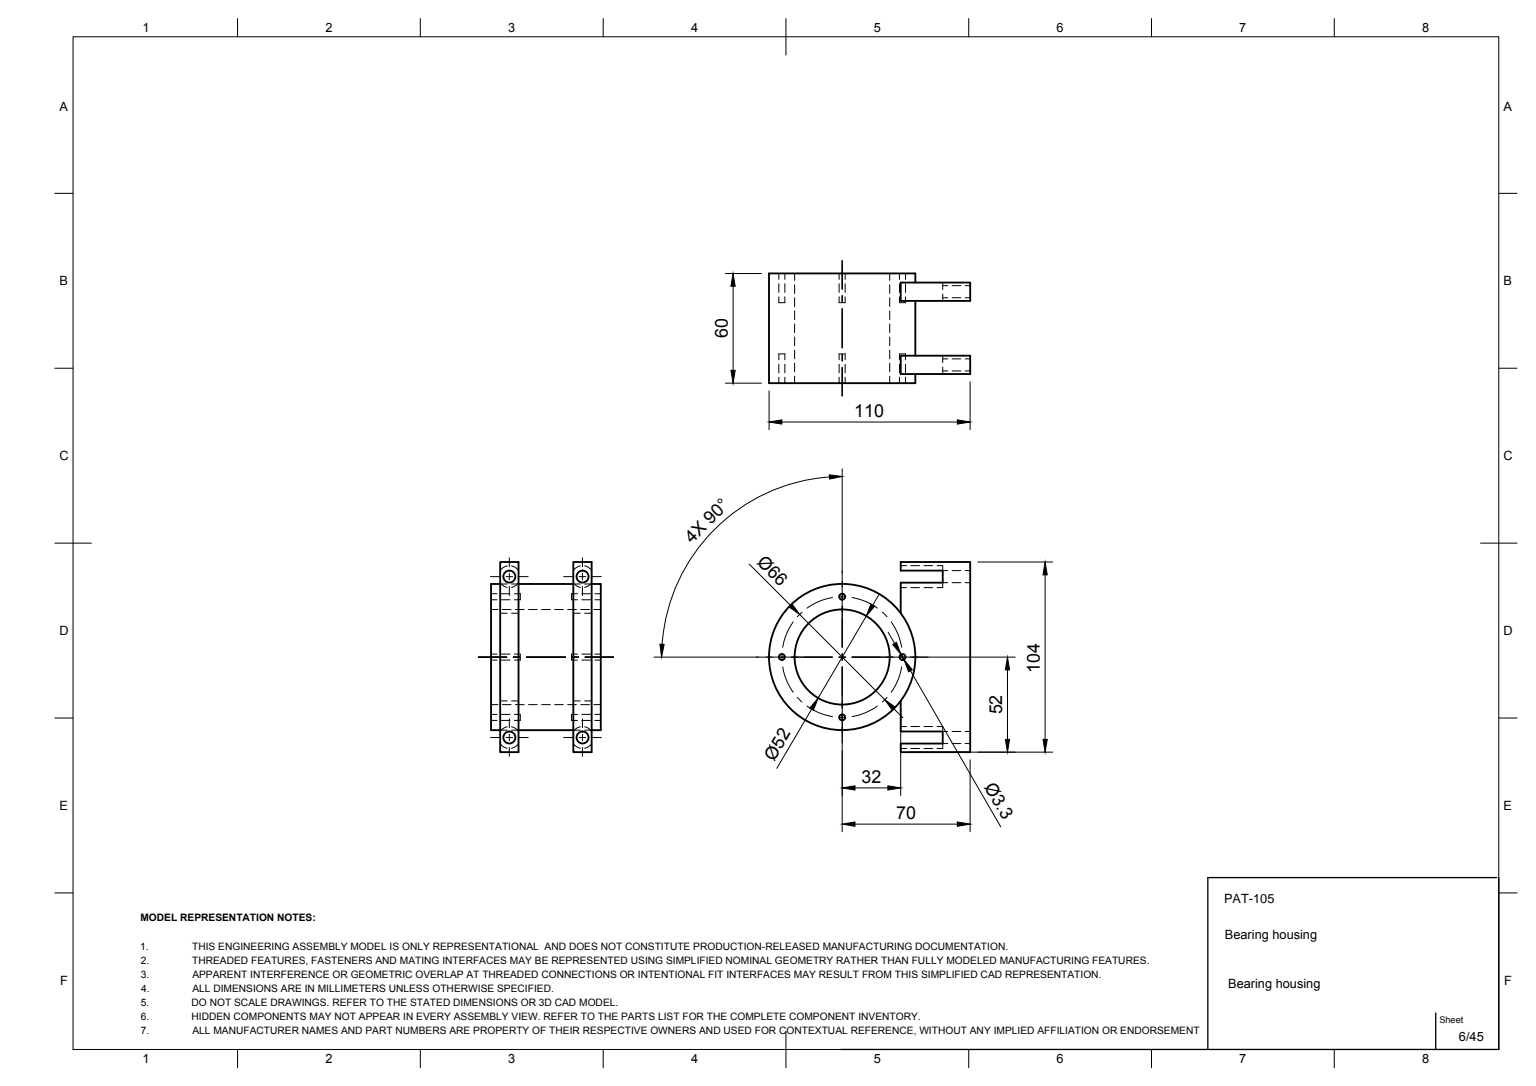
ISO-10303-21;
HEADER;
/* Generated by software containing ST-Developer
 * from STEP Tools, Inc. (www.steptools.com) 
 */

FILE_DESCRIPTION(
/* description */ ('Torque wrench calibration arm'),
/* implementation_level */ '2;1');

FILE_NAME(
/* name */ 'Bearing housing.step',
/* time_stamp */ '2026-10-28T03:24:52-07:00',
/* author */ (''),
/* organization */ (''),
/* preprocessor_version */ 'ST-DEVELOPER v20.2',
/* originating_system */ 'Autodesk Translation Framework v15.17.0.0',
/* authorisation */ '');

FILE_SCHEMA (('AUTOMOTIVE_DESIGN { 1 0 10303 214 3 1 1 }'));
ENDSEC;

DATA;
#10=MECHANICAL_DESIGN_GEOMETRIC_PRESENTATION_REPRESENTATION('',(#427),#12783);
#353=SHAPE_REPRESENTATION_RELATIONSHIP('SRR','None',#12934,#390);
#390=ADVANCED_BREP_SHAPE_REPRESENTATION('',(#481),#12743);
#427=STYLED_ITEM('',(#13212),#481);
#481=MANIFOLD_SOLID_BREP('Body1',#6496);
#539=FACE_BOUND('',#1307,.T.);
#540=FACE_BOUND('',#1311,.T.);
#541=FACE_BOUND('',#1315,.T.);
#542=FACE_BOUND('',#1319,.T.);
#543=FACE_BOUND('',#1336,.T.);
#544=FACE_BOUND('',#1337,.T.);
#545=FACE_BOUND('',#1342,.T.);
#546=FACE_BOUND('',#1343,.T.);
#547=FACE_BOUND('',#1348,.T.);
#548=FACE_BOUND('',#1349,.T.);
#549=FACE_BOUND('',#1351,.T.);
#550=FACE_BOUND('',#1352,.T.);
#551=FACE_BOUND('',#1353,.T.);
#552=FACE_BOUND('',#1354,.T.);
#553=FACE_BOUND('',#1355,.T.);
#554=FACE_BOUND('',#1357,.T.);
#555=FACE_BOUND('',#1358,.T.);
#556=FACE_BOUND('',#1359,.T.);
#557=FACE_BOUND('',#1360,.T.);
#558=FACE_BOUND('',#1361,.T.);
#658=PLANE('',#6985);
#659=PLANE('',#6989);
#660=PLANE('',#6993);
#661=PLANE('',#6997);
#662=PLANE('',#7001);
#663=PLANE('',#7005);
#664=PLANE('',#7009);
#665=PLANE('',#7013);
#666=PLANE('',#7020);
#667=PLANE('',#7028);
#668=PLANE('',#7036);
#669=PLANE('',#7044);
#670=PLANE('',#7046);
#671=PLANE('',#7047);
#672=PLANE('',#7048);
#673=PLANE('',#7049);
#674=PLANE('',#7050);
#675=PLANE('',#7052);
#676=PLANE('',#7053);
#677=PLANE('',#7054);
#678=PLANE('',#7056);
#679=PLANE('',#7057);
#680=PLANE('',#7066);
#681=PLANE('',#7067);
#682=PLANE('',#7068);
#683=PLANE('',#7069);
#684=PLANE('',#7071);
#685=PLANE('',#7072);
#686=PLANE('',#7073);
#687=PLANE('',#7074);
#688=PLANE('',#7082);
#689=PLANE('',#7083);
#885=FACE_OUTER_BOUND('',#1288,.T.);
#886=FACE_OUTER_BOUND('',#1289,.T.);
#887=FACE_OUTER_BOUND('',#1290,.T.);
#888=FACE_OUTER_BOUND('',#1291,.T.);
#889=FACE_OUTER_BOUND('',#1292,.T.);
#890=FACE_OUTER_BOUND('',#1293,.T.);
#891=FACE_OUTER_BOUND('',#1294,.T.);
#892=FACE_OUTER_BOUND('',#1295,.T.);
#893=FACE_OUTER_BOUND('',#1296,.T.);
#894=FACE_OUTER_BOUND('',#1297,.T.);
#895=FACE_OUTER_BOUND('',#1298,.T.);
#896=FACE_OUTER_BOUND('',#1299,.T.);
#897=FACE_OUTER_BOUND('',#1300,.T.);
#898=FACE_OUTER_BOUND('',#1301,.T.);
#899=FACE_OUTER_BOUND('',#1302,.T.);
#900=FACE_OUTER_BOUND('',#1303,.T.);
#901=FACE_OUTER_BOUND('',#1304,.T.);
#902=FACE_OUTER_BOUND('',#1305,.T.);
#903=FACE_OUTER_BOUND('',#1306,.T.);
#904=FACE_OUTER_BOUND('',#1308,.T.);
#905=FACE_OUTER_BOUND('',#1309,.T.);
#906=FACE_OUTER_BOUND('',#1310,.T.);
#907=FACE_OUTER_BOUND('',#1312,.T.);
#908=FACE_OUTER_BOUND('',#1313,.T.);
#909=FACE_OUTER_BOUND('',#1314,.T.);
#910=FACE_OUTER_BOUND('',#1316,.T.);
#911=FACE_OUTER_BOUND('',#1317,.T.);
#912=FACE_OUTER_BOUND('',#1318,.T.);
#913=FACE_OUTER_BOUND('',#1320,.T.);
#914=FACE_OUTER_BOUND('',#1321,.T.);
#915=FACE_OUTER_BOUND('',#1322,.T.);
#916=FACE_OUTER_BOUND('',#1323,.T.);
#917=FACE_OUTER_BOUND('',#1324,.T.);
#918=FACE_OUTER_BOUND('',#1325,.T.);
#919=FACE_OUTER_BOUND('',#1326,.T.);
#920=FACE_OUTER_BOUND('',#1327,.T.);
#921=FACE_OUTER_BOUND('',#1328,.T.);
#922=FACE_OUTER_BOUND('',#1329,.T.);
#923=FACE_OUTER_BOUND('',#1330,.T.);
#924=FACE_OUTER_BOUND('',#1331,.T.);
#925=FACE_OUTER_BOUND('',#1332,.T.);
#926=FACE_OUTER_BOUND('',#1333,.T.);
#927=FACE_OUTER_BOUND('',#1334,.T.);
#928=FACE_OUTER_BOUND('',#1335,.T.);
#929=FACE_OUTER_BOUND('',#1338,.T.);
#930=FACE_OUTER_BOUND('',#1339,.T.);
#931=FACE_OUTER_BOUND('',#1340,.T.);
#932=FACE_OUTER_BOUND('',#1341,.T.);
#933=FACE_OUTER_BOUND('',#1344,.T.);
#934=FACE_OUTER_BOUND('',#1345,.T.);
#935=FACE_OUTER_BOUND('',#1346,.T.);
#936=FACE_OUTER_BOUND('',#1347,.T.);
#937=FACE_OUTER_BOUND('',#1350,.T.);
#938=FACE_OUTER_BOUND('',#1356,.T.);
#1288=EDGE_LOOP('',(#4399,#4400,#4401,#4402));
#1289=EDGE_LOOP('',(#4403));
#1290=EDGE_LOOP('',(#4404,#4405,#4406,#4407));
#1291=EDGE_LOOP('',(#4408));
#1292=EDGE_LOOP('',(#4409,#4410,#4411,#4412));
#1293=EDGE_LOOP('',(#4413));
#1294=EDGE_LOOP('',(#4414,#4415,#4416,#4417));
#1295=EDGE_LOOP('',(#4418));
#1296=EDGE_LOOP('',(#4419,#4420,#4421,#4422));
#1297=EDGE_LOOP('',(#4423));
#1298=EDGE_LOOP('',(#4424,#4425,#4426,#4427));
#1299=EDGE_LOOP('',(#4428));
#1300=EDGE_LOOP('',(#4429,#4430,#4431,#4432));
#1301=EDGE_LOOP('',(#4433));
#1302=EDGE_LOOP('',(#4434,#4435,#4436,#4437));
#1303=EDGE_LOOP('',(#4438));
#1304=EDGE_LOOP('',(#4439,#4440,#4441,#4442));
#1305=EDGE_LOOP('',(#4443,#4444,#4445,#4446));
#1306=EDGE_LOOP('',(#4447,#4448,#4449,#4450));
#1307=EDGE_LOOP('',(#4451));
#1308=EDGE_LOOP('',(#4452,#4453,#4454,#4455));
#1309=EDGE_LOOP('',(#4456,#4457,#4458,#4459));
#1310=EDGE_LOOP('',(#4460,#4461,#4462,#4463));
#1311=EDGE_LOOP('',(#4464));
#1312=EDGE_LOOP('',(#4465,#4466,#4467,#4468));
#1313=EDGE_LOOP('',(#4469,#4470,#4471,#4472));
#1314=EDGE_LOOP('',(#4473,#4474,#4475,#4476));
#1315=EDGE_LOOP('',(#4477));
#1316=EDGE_LOOP('',(#4478,#4479,#4480,#4481));
#1317=EDGE_LOOP('',(#4482,#4483,#4484,#4485));
#1318=EDGE_LOOP('',(#4486,#4487,#4488,#4489));
#1319=EDGE_LOOP('',(#4490));
#1320=EDGE_LOOP('',(#4491,#4492,#4493,#4494));
#1321=EDGE_LOOP('',(#4495,#4496,#4497,#4498));
#1322=EDGE_LOOP('',(#4499,#4500,#4501,#4502));
#1323=EDGE_LOOP('',(#4503,#4504,#4505,#4506));
#1324=EDGE_LOOP('',(#4507,#4508,#4509,#4510,#4511,#4512,#4513,#4514,#4515,
#4516,#4517,#4518,#4519,#4520));
#1325=EDGE_LOOP('',(#4521,#4522,#4523,#4524));
#1326=EDGE_LOOP('',(#4525,#4526,#4527,#4528));
#1327=EDGE_LOOP('',(#4529,#4530,#4531,#4532,#4533,#4534,#4535,#4536,#4537,
#4538,#4539,#4540,#4541,#4542));
#1328=EDGE_LOOP('',(#4543,#4544,#4545,#4546));
#1329=EDGE_LOOP('',(#4547,#4548,#4549,#4550));
#1330=EDGE_LOOP('',(#4551,#4552,#4553,#4554));
#1331=EDGE_LOOP('',(#4555,#4556,#4557,#4558));
#1332=EDGE_LOOP('',(#4559,#4560,#4561,#4562));
#1333=EDGE_LOOP('',(#4563,#4564,#4565,#4566));
#1334=EDGE_LOOP('',(#4567,#4568,#4569,#4570));
#1335=EDGE_LOOP('',(#4571,#4572,#4573,#4574));
#1336=EDGE_LOOP('',(#4575));
#1337=EDGE_LOOP('',(#4576));
#1338=EDGE_LOOP('',(#4577,#4578,#4579,#4580));
#1339=EDGE_LOOP('',(#4581,#4582,#4583,#4584,#4585,#4586,#4587,#4588,#4589,
#4590,#4591,#4592,#4593,#4594));
#1340=EDGE_LOOP('',(#4595,#4596,#4597,#4598));
#1341=EDGE_LOOP('',(#4599,#4600,#4601,#4602));
#1342=EDGE_LOOP('',(#4603));
#1343=EDGE_LOOP('',(#4604));
#1344=EDGE_LOOP('',(#4605,#4606,#4607,#4608));
#1345=EDGE_LOOP('',(#4609,#4610,#4611,#4612,#4613,#4614,#4615,#4616,#4617,
#4618,#4619,#4620,#4621,#4622));
#1346=EDGE_LOOP('',(#4623,#4624,#4625,#4626));
#1347=EDGE_LOOP('',(#4627,#4628,#4629,#4630));
#1348=EDGE_LOOP('',(#4631,#4632,#4633,#4634));
#1349=EDGE_LOOP('',(#4635,#4636,#4637,#4638));
#1350=EDGE_LOOP('',(#4639));
#1351=EDGE_LOOP('',(#4640));
#1352=EDGE_LOOP('',(#4641));
#1353=EDGE_LOOP('',(#4642));
#1354=EDGE_LOOP('',(#4643));
#1355=EDGE_LOOP('',(#4644));
#1356=EDGE_LOOP('',(#4645));
#1357=EDGE_LOOP('',(#4646));
#1358=EDGE_LOOP('',(#4647));
#1359=EDGE_LOOP('',(#4648));
#1360=EDGE_LOOP('',(#4649));
#1361=EDGE_LOOP('',(#4650));
#1802=LINE('',#9983,#2217);
#1803=LINE('',#9990,#2218);
#1804=LINE('',#9997,#2219);
#1805=LINE('',#10004,#2220);
#1806=LINE('',#10011,#2221);
#1807=LINE('',#10018,#2222);
#1808=LINE('',#10025,#2223);
#1809=LINE('',#10032,#2224);
#1810=LINE('',#10038,#2225);
#1811=LINE('',#10042,#2226);
#1812=LINE('',#10047,#2227);
#1813=LINE('',#10051,#2228);
#1814=LINE('',#10054,#2229);
#1815=LINE('',#10055,#2230);
#1816=LINE('',#10061,#2231);
#1817=LINE('',#10065,#2232);
#1818=LINE('',#10070,#2233);
#1819=LINE('',#10074,#2234);
#1820=LINE('',#10077,#2235);
#1821=LINE('',#10078,#2236);
#1822=LINE('',#10084,#2237);
#1823=LINE('',#10088,#2238);
#1824=LINE('',#10093,#2239);
#1825=LINE('',#10097,#2240);
#1826=LINE('',#10100,#2241);
#1827=LINE('',#10101,#2242);
#1828=LINE('',#10107,#2243);
#1829=LINE('',#10111,#2244);
#1830=LINE('',#10116,#2245);
#1831=LINE('',#10120,#2246);
#1832=LINE('',#10123,#2247);
#1833=LINE('',#10124,#2248);
#1834=LINE('',#10129,#2249);
#1835=LINE('',#10131,#2250);
#1836=LINE('',#10132,#2251);
#1837=LINE('',#10135,#2252);
#1838=LINE('',#10137,#2253);
#1839=LINE('',#10138,#2254);
#1840=LINE('',#10141,#2255);
#1841=LINE('',#10143,#2256);
#1842=LINE('',#10144,#2257);
#1843=LINE('',#10147,#2258);
#1844=LINE('',#10149,#2259);
#1845=LINE('',#10150,#2260);
#1846=LINE('',#10153,#2261);
#1847=LINE('',#10155,#2262);
#1848=LINE('',#10157,#2263);
#1849=LINE('',#10158,#2264);
#1850=LINE('',#10160,#2265);
#1851=LINE('',#10164,#2266);
#1852=LINE('',#10165,#2267);
#1853=LINE('',#10168,#2268);
#1854=LINE('',#10169,#2269);
#1855=LINE('',#10173,#2270);
#1856=LINE('',#10175,#2271);
#1857=LINE('',#10177,#2272);
#1858=LINE('',#10179,#2273);
#1859=LINE('',#10180,#2274);
#1860=LINE('',#10183,#2275);
#1861=LINE('',#10184,#2276);
#1862=LINE('',#10187,#2277);
#1863=LINE('',#10188,#2278);
#1864=LINE('',#10192,#2279);
#1865=LINE('',#10196,#2280);
#1866=LINE('',#10200,#2281);
#1867=LINE('',#10204,#2282);
#1868=LINE('',#10207,#2283);
#1869=LINE('',#10208,#2284);
#1870=LINE('',#10211,#2285);
#1871=LINE('',#10212,#2286);
#1872=LINE('',#10214,#2287);
#1873=LINE('',#10219,#2288);
#1874=LINE('',#10220,#2289);
#1875=LINE('',#10223,#2290);
#1876=LINE('',#10224,#2291);
#1877=LINE('',#10226,#2292);
#1878=LINE('',#10233,#2293);
#1879=LINE('',#10239,#2294);
#2217=VECTOR('',#7874,0.165);
#2218=VECTOR('',#7883,0.165);
#2219=VECTOR('',#7892,0.165);
#2220=VECTOR('',#7901,0.165);
#2221=VECTOR('',#7910,0.165);
#2222=VECTOR('',#7919,0.165);
#2223=VECTOR('',#7928,0.165);
#2224=VECTOR('',#7937,0.165);
#2225=VECTOR('',#7944,1.);
#2226=VECTOR('',#7947,1.);
#2227=VECTOR('',#7952,1.);
#2228=VECTOR('',#7955,1.);
#2229=VECTOR('',#7960,1.);
#2230=VECTOR('',#7961,1.);
#2231=VECTOR('',#7966,1.);
#2232=VECTOR('',#7969,1.);
#2233=VECTOR('',#7974,1.);
#2234=VECTOR('',#7977,1.);
#2235=VECTOR('',#7982,1.);
#2236=VECTOR('',#7983,1.);
#2237=VECTOR('',#7988,1.);
#2238=VECTOR('',#7991,1.);
#2239=VECTOR('',#7996,1.);
#2240=VECTOR('',#7999,1.);
#2241=VECTOR('',#8004,1.);
#2242=VECTOR('',#8005,1.);
#2243=VECTOR('',#8010,1.);
#2244=VECTOR('',#8013,1.);
#2245=VECTOR('',#8018,1.);
#2246=VECTOR('',#8021,1.);
#2247=VECTOR('',#8026,1.);
#2248=VECTOR('',#8027,1.);
#2249=VECTOR('',#8032,1.);
#2250=VECTOR('',#8033,1.);
#2251=VECTOR('',#8034,1.);
#2252=VECTOR('',#8037,1.);
#2253=VECTOR('',#8038,1.);
#2254=VECTOR('',#8039,1.);
#2255=VECTOR('',#8042,1.);
#2256=VECTOR('',#8043,1.);
#2257=VECTOR('',#8044,1.);
#2258=VECTOR('',#8047,1.);
#2259=VECTOR('',#8048,1.);
#2260=VECTOR('',#8049,1.);
#2261=VECTOR('',#8052,1.);
#2262=VECTOR('',#8053,1.);
#2263=VECTOR('',#8054,1.);
#2264=VECTOR('',#8055,1.);
#2265=VECTOR('',#8056,1.);
#2266=VECTOR('',#8061,1.);
#2267=VECTOR('',#8062,1.);
#2268=VECTOR('',#8065,1.);
#2269=VECTOR('',#8066,1.);
#2270=VECTOR('',#8071,1.);
#2271=VECTOR('',#8072,1.);
#2272=VECTOR('',#8073,1.);
#2273=VECTOR('',#8074,1.);
#2274=VECTOR('',#8075,1.);
#2275=VECTOR('',#8078,1.);
#2276=VECTOR('',#8079,1.);
#2277=VECTOR('',#8082,1.);
#2278=VECTOR('',#8083,1.);
#2279=VECTOR('',#8088,0.33);
#2280=VECTOR('',#8093,0.33);
#2281=VECTOR('',#8098,0.33);
#2282=VECTOR('',#8103,0.33);
#2283=VECTOR('',#8106,1.);
#2284=VECTOR('',#8107,1.);
#2285=VECTOR('',#8110,1.);
#2286=VECTOR('',#8111,1.);
#2287=VECTOR('',#8114,1.);
#2288=VECTOR('',#8121,1.);
#2289=VECTOR('',#8122,1.);
#2290=VECTOR('',#8125,1.);
#2291=VECTOR('',#8126,1.);
#2292=VECTOR('',#8129,1.);
#2293=VECTOR('',#8138,2.6);
#2294=VECTOR('',#8145,4.);
#2624=CIRCLE('',#6983,0.165);
#2625=CIRCLE('',#6984,0.165);
#2626=CIRCLE('',#6987,0.165);
#2627=CIRCLE('',#6988,0.165);
#2628=CIRCLE('',#6991,0.165);
#2629=CIRCLE('',#6992,0.165);
#2630=CIRCLE('',#6995,0.165);
#2631=CIRCLE('',#6996,0.165);
#2632=CIRCLE('',#6999,0.165);
#2633=CIRCLE('',#7000,0.165);
#2634=CIRCLE('',#7003,0.165);
#2635=CIRCLE('',#7004,0.165);
#2636=CIRCLE('',#7007,0.165);
#2637=CIRCLE('',#7008,0.165);
#2638=CIRCLE('',#7011,0.165);
#2639=CIRCLE('',#7012,0.165);
#2640=CIRCLE('',#7015,0.6);
#2641=CIRCLE('',#7016,0.6);
#2642=CIRCLE('',#7018,0.6);
#2643=CIRCLE('',#7019,0.6);
#2644=CIRCLE('',#7021,0.33);
#2645=CIRCLE('',#7023,0.6);
#2646=CIRCLE('',#7024,0.6);
#2647=CIRCLE('',#7026,0.6);
#2648=CIRCLE('',#7027,0.6);
#2649=CIRCLE('',#7029,0.33);
#2650=CIRCLE('',#7031,0.6);
#2651=CIRCLE('',#7032,0.6);
#2652=CIRCLE('',#7034,0.6);
#2653=CIRCLE('',#7035,0.6);
#2654=CIRCLE('',#7037,0.33);
#2655=CIRCLE('',#7039,0.6);
#2656=CIRCLE('',#7040,0.6);
#2657=CIRCLE('',#7042,0.6);
#2658=CIRCLE('',#7043,0.6);
#2659=CIRCLE('',#7045,0.33);
#2660=CIRCLE('',#7051,4.);
#2661=CIRCLE('',#7055,4.);
#2662=CIRCLE('',#7059,0.33);
#2663=CIRCLE('',#7061,0.33);
#2664=CIRCLE('',#7063,0.33);
#2665=CIRCLE('',#7065,0.33);
#2666=CIRCLE('',#7070,4.);
#2667=CIRCLE('',#7075,4.);
#2668=CIRCLE('',#7077,2.6);
#2669=CIRCLE('',#7078,2.6);
#2670=CIRCLE('',#7080,4.);
#2671=CIRCLE('',#7081,4.);
#2987=VERTEX_POINT('',#9980);
#2988=VERTEX_POINT('',#9982);
#2989=VERTEX_POINT('',#9987);
#2990=VERTEX_POINT('',#9989);
#2991=VERTEX_POINT('',#9994);
#2992=VERTEX_POINT('',#9996);
#2993=VERTEX_POINT('',#10001);
#2994=VERTEX_POINT('',#10003);
#2995=VERTEX_POINT('',#10008);
#2996=VERTEX_POINT('',#10010);
#2997=VERTEX_POINT('',#10015);
#2998=VERTEX_POINT('',#10017);
#2999=VERTEX_POINT('',#10022);
#3000=VERTEX_POINT('',#10024);
#3001=VERTEX_POINT('',#10029);
#3002=VERTEX_POINT('',#10031);
#3003=VERTEX_POINT('',#10036);
#3004=VERTEX_POINT('',#10037);
#3005=VERTEX_POINT('',#10039);
#3006=VERTEX_POINT('',#10041);
#3007=VERTEX_POINT('',#10045);
#3008=VERTEX_POINT('',#10046);
#3009=VERTEX_POINT('',#10048);
#3010=VERTEX_POINT('',#10050);
#3011=VERTEX_POINT('',#10056);
#3012=VERTEX_POINT('',#10059);
#3013=VERTEX_POINT('',#10060);
#3014=VERTEX_POINT('',#10062);
#3015=VERTEX_POINT('',#10064);
#3016=VERTEX_POINT('',#10068);
#3017=VERTEX_POINT('',#10069);
#3018=VERTEX_POINT('',#10071);
#3019=VERTEX_POINT('',#10073);
#3020=VERTEX_POINT('',#10079);
#3021=VERTEX_POINT('',#10082);
#3022=VERTEX_POINT('',#10083);
#3023=VERTEX_POINT('',#10085);
#3024=VERTEX_POINT('',#10087);
#3025=VERTEX_POINT('',#10091);
#3026=VERTEX_POINT('',#10092);
#3027=VERTEX_POINT('',#10094);
#3028=VERTEX_POINT('',#10096);
#3029=VERTEX_POINT('',#10102);
#3030=VERTEX_POINT('',#10105);
#3031=VERTEX_POINT('',#10106);
#3032=VERTEX_POINT('',#10108);
#3033=VERTEX_POINT('',#10110);
#3034=VERTEX_POINT('',#10114);
#3035=VERTEX_POINT('',#10115);
#3036=VERTEX_POINT('',#10117);
#3037=VERTEX_POINT('',#10119);
#3038=VERTEX_POINT('',#10125);
#3039=VERTEX_POINT('',#10128);
#3040=VERTEX_POINT('',#10130);
#3041=VERTEX_POINT('',#10134);
#3042=VERTEX_POINT('',#10136);
#3043=VERTEX_POINT('',#10140);
#3044=VERTEX_POINT('',#10142);
#3045=VERTEX_POINT('',#10146);
#3046=VERTEX_POINT('',#10148);
#3047=VERTEX_POINT('',#10152);
#3048=VERTEX_POINT('',#10154);
#3049=VERTEX_POINT('',#10156);
#3050=VERTEX_POINT('',#10159);
#3051=VERTEX_POINT('',#10163);
#3052=VERTEX_POINT('',#10167);
#3053=VERTEX_POINT('',#10171);
#3054=VERTEX_POINT('',#10174);
#3055=VERTEX_POINT('',#10176);
#3056=VERTEX_POINT('',#10178);
#3057=VERTEX_POINT('',#10182);
#3058=VERTEX_POINT('',#10186);
#3059=VERTEX_POINT('',#10190);
#3060=VERTEX_POINT('',#10194);
#3061=VERTEX_POINT('',#10198);
#3062=VERTEX_POINT('',#10202);
#3063=VERTEX_POINT('',#10206);
#3064=VERTEX_POINT('',#10210);
#3065=VERTEX_POINT('',#10218);
#3066=VERTEX_POINT('',#10222);
#3067=VERTEX_POINT('',#10230);
#3068=VERTEX_POINT('',#10232);
#3069=VERTEX_POINT('',#10236);
#3070=VERTEX_POINT('',#10238);
#3557=EDGE_CURVE('',#2987,#2987,#2624,.T.);
#3558=EDGE_CURVE('',#2987,#2988,#1802,.T.);
#3559=EDGE_CURVE('',#2988,#2988,#2625,.T.);
#3560=EDGE_CURVE('',#2989,#2989,#2626,.T.);
#3561=EDGE_CURVE('',#2989,#2990,#1803,.T.);
#3562=EDGE_CURVE('',#2990,#2990,#2627,.T.);
#3563=EDGE_CURVE('',#2991,#2991,#2628,.T.);
#3564=EDGE_CURVE('',#2991,#2992,#1804,.T.);
#3565=EDGE_CURVE('',#2992,#2992,#2629,.T.);
#3566=EDGE_CURVE('',#2993,#2993,#2630,.T.);
#3567=EDGE_CURVE('',#2993,#2994,#1805,.T.);
#3568=EDGE_CURVE('',#2994,#2994,#2631,.T.);
#3569=EDGE_CURVE('',#2995,#2995,#2632,.T.);
#3570=EDGE_CURVE('',#2995,#2996,#1806,.T.);
#3571=EDGE_CURVE('',#2996,#2996,#2633,.T.);
#3572=EDGE_CURVE('',#2997,#2997,#2634,.T.);
#3573=EDGE_CURVE('',#2997,#2998,#1807,.T.);
#3574=EDGE_CURVE('',#2998,#2998,#2635,.T.);
#3575=EDGE_CURVE('',#2999,#2999,#2636,.T.);
#3576=EDGE_CURVE('',#2999,#3000,#1808,.T.);
#3577=EDGE_CURVE('',#3000,#3000,#2637,.T.);
#3578=EDGE_CURVE('',#3001,#3001,#2638,.T.);
#3579=EDGE_CURVE('',#3001,#3002,#1809,.T.);
#3580=EDGE_CURVE('',#3002,#3002,#2639,.T.);
#3581=EDGE_CURVE('',#3003,#3004,#1810,.T.);
#3582=EDGE_CURVE('',#3005,#3003,#2640,.T.);
#3583=EDGE_CURVE('',#3006,#3005,#1811,.T.);
#3584=EDGE_CURVE('',#3004,#3006,#2641,.T.);
#3585=EDGE_CURVE('',#3007,#3008,#1812,.T.);
#3586=EDGE_CURVE('',#3009,#3007,#2642,.T.);
#3587=EDGE_CURVE('',#3010,#3009,#1813,.T.);
#3588=EDGE_CURVE('',#3008,#3010,#2643,.T.);
#3589=EDGE_CURVE('',#3004,#3007,#1814,.T.);
#3590=EDGE_CURVE('',#3009,#3006,#1815,.T.);
#3591=EDGE_CURVE('',#3011,#3011,#2644,.T.);
#3592=EDGE_CURVE('',#3012,#3013,#1816,.T.);
#3593=EDGE_CURVE('',#3014,#3012,#2645,.T.);
#3594=EDGE_CURVE('',#3015,#3014,#1817,.T.);
#3595=EDGE_CURVE('',#3013,#3015,#2646,.T.);
#3596=EDGE_CURVE('',#3016,#3017,#1818,.T.);
#3597=EDGE_CURVE('',#3018,#3016,#2647,.T.);
#3598=EDGE_CURVE('',#3019,#3018,#1819,.T.);
#3599=EDGE_CURVE('',#3017,#3019,#2648,.T.);
#3600=EDGE_CURVE('',#3013,#3016,#1820,.T.);
#3601=EDGE_CURVE('',#3018,#3015,#1821,.T.);
#3602=EDGE_CURVE('',#3020,#3020,#2649,.T.);
#3603=EDGE_CURVE('',#3021,#3022,#1822,.T.);
#3604=EDGE_CURVE('',#3023,#3021,#2650,.T.);
#3605=EDGE_CURVE('',#3024,#3023,#1823,.T.);
#3606=EDGE_CURVE('',#3022,#3024,#2651,.T.);
#3607=EDGE_CURVE('',#3025,#3026,#1824,.T.);
#3608=EDGE_CURVE('',#3027,#3025,#2652,.T.);
#3609=EDGE_CURVE('',#3028,#3027,#1825,.T.);
#3610=EDGE_CURVE('',#3026,#3028,#2653,.T.);
#3611=EDGE_CURVE('',#3022,#3025,#1826,.T.);
#3612=EDGE_CURVE('',#3027,#3024,#1827,.T.);
#3613=EDGE_CURVE('',#3029,#3029,#2654,.T.);
#3614=EDGE_CURVE('',#3030,#3031,#1828,.T.);
#3615=EDGE_CURVE('',#3032,#3030,#2655,.T.);
#3616=EDGE_CURVE('',#3033,#3032,#1829,.T.);
#3617=EDGE_CURVE('',#3031,#3033,#2656,.T.);
#3618=EDGE_CURVE('',#3034,#3035,#1830,.T.);
#3619=EDGE_CURVE('',#3036,#3034,#2657,.T.);
#3620=EDGE_CURVE('',#3037,#3036,#1831,.T.);
#3621=EDGE_CURVE('',#3035,#3037,#2658,.T.);
#3622=EDGE_CURVE('',#3031,#3034,#1832,.T.);
#3623=EDGE_CURVE('',#3036,#3033,#1833,.T.);
#3624=EDGE_CURVE('',#3038,#3038,#2659,.T.);
#3625=EDGE_CURVE('',#3039,#3003,#1834,.T.);
#3626=EDGE_CURVE('',#3039,#3040,#1835,.T.);
#3627=EDGE_CURVE('',#3005,#3040,#1836,.T.);
#3628=EDGE_CURVE('',#3041,#3010,#1837,.T.);
#3629=EDGE_CURVE('',#3042,#3041,#1838,.T.);
#3630=EDGE_CURVE('',#3008,#3042,#1839,.T.);
#3631=EDGE_CURVE('',#3043,#3012,#1840,.T.);
#3632=EDGE_CURVE('',#3044,#3043,#1841,.T.);
#3633=EDGE_CURVE('',#3014,#3044,#1842,.T.);
#3634=EDGE_CURVE('',#3045,#3019,#1843,.T.);
#3635=EDGE_CURVE('',#3046,#3045,#1844,.T.);
#3636=EDGE_CURVE('',#3017,#3046,#1845,.T.);
#3637=EDGE_CURVE('',#3040,#3047,#1846,.T.);
#3638=EDGE_CURVE('',#3047,#3048,#1847,.T.);
#3639=EDGE_CURVE('',#3048,#3049,#1848,.T.);
#3640=EDGE_CURVE('',#3049,#3028,#1849,.T.);
#3641=EDGE_CURVE('',#3023,#3050,#1850,.T.);
#3642=EDGE_CURVE('',#3041,#3050,#2660,.T.);
#3643=EDGE_CURVE('',#3051,#3021,#1851,.T.);
#3644=EDGE_CURVE('',#3050,#3051,#1852,.T.);
#3645=EDGE_CURVE('',#3052,#3049,#1853,.T.);
#3646=EDGE_CURVE('',#3026,#3052,#1854,.T.);
#3647=EDGE_CURVE('',#3053,#3044,#2661,.T.);
#3648=EDGE_CURVE('',#3053,#3037,#1855,.T.);
#3649=EDGE_CURVE('',#3032,#3054,#1856,.T.);
#3650=EDGE_CURVE('',#3054,#3055,#1857,.T.);
#3651=EDGE_CURVE('',#3055,#3056,#1858,.T.);
#3652=EDGE_CURVE('',#3056,#3045,#1859,.T.);
#3653=EDGE_CURVE('',#3057,#3030,#1860,.T.);
#3654=EDGE_CURVE('',#3057,#3054,#1861,.T.);
#3655=EDGE_CURVE('',#3058,#3053,#1862,.T.);
#3656=EDGE_CURVE('',#3035,#3058,#1863,.T.);
#3657=EDGE_CURVE('',#3059,#3059,#2662,.T.);
#3658=EDGE_CURVE('',#3059,#3011,#1864,.T.);
#3659=EDGE_CURVE('',#3060,#3060,#2663,.T.);
#3660=EDGE_CURVE('',#3060,#3020,#1865,.T.);
#3661=EDGE_CURVE('',#3061,#3061,#2664,.T.);
#3662=EDGE_CURVE('',#3061,#3029,#1866,.T.);
#3663=EDGE_CURVE('',#3062,#3062,#2665,.T.);
#3664=EDGE_CURVE('',#3062,#3038,#1867,.T.);
#3665=EDGE_CURVE('',#3046,#3063,#1868,.T.);
#3666=EDGE_CURVE('',#3063,#3056,#1869,.T.);
#3667=EDGE_CURVE('',#3063,#3064,#1870,.T.);
#3668=EDGE_CURVE('',#3064,#3055,#1871,.T.);
#3669=EDGE_CURVE('',#3064,#3057,#1872,.T.);
#3670=EDGE_CURVE('',#3043,#3058,#2666,.T.);
#3671=EDGE_CURVE('',#3052,#3065,#1873,.T.);
#3672=EDGE_CURVE('',#3065,#3048,#1874,.T.);
#3673=EDGE_CURVE('',#3065,#3066,#1875,.T.);
#3674=EDGE_CURVE('',#3066,#3047,#1876,.T.);
#3675=EDGE_CURVE('',#3066,#3039,#1877,.T.);
#3676=EDGE_CURVE('',#3051,#3042,#2667,.T.);
#3677=EDGE_CURVE('',#3067,#3067,#2668,.T.);
#3678=EDGE_CURVE('',#3067,#3068,#1878,.T.);
#3679=EDGE_CURVE('',#3068,#3068,#2669,.T.);
#3680=EDGE_CURVE('',#3069,#3069,#2670,.T.);
#3681=EDGE_CURVE('',#3069,#3070,#1879,.T.);
#3682=EDGE_CURVE('',#3070,#3070,#2671,.T.);
#4399=ORIENTED_EDGE('',*,*,#3557,.F.);
#4400=ORIENTED_EDGE('',*,*,#3558,.T.);
#4401=ORIENTED_EDGE('',*,*,#3559,.F.);
#4402=ORIENTED_EDGE('',*,*,#3558,.F.);
#4403=ORIENTED_EDGE('',*,*,#3557,.T.);
#4404=ORIENTED_EDGE('',*,*,#3560,.F.);
#4405=ORIENTED_EDGE('',*,*,#3561,.T.);
#4406=ORIENTED_EDGE('',*,*,#3562,.F.);
#4407=ORIENTED_EDGE('',*,*,#3561,.F.);
#4408=ORIENTED_EDGE('',*,*,#3560,.T.);
#4409=ORIENTED_EDGE('',*,*,#3563,.F.);
#4410=ORIENTED_EDGE('',*,*,#3564,.T.);
#4411=ORIENTED_EDGE('',*,*,#3565,.F.);
#4412=ORIENTED_EDGE('',*,*,#3564,.F.);
#4413=ORIENTED_EDGE('',*,*,#3563,.T.);
#4414=ORIENTED_EDGE('',*,*,#3566,.F.);
#4415=ORIENTED_EDGE('',*,*,#3567,.T.);
#4416=ORIENTED_EDGE('',*,*,#3568,.F.);
#4417=ORIENTED_EDGE('',*,*,#3567,.F.);
#4418=ORIENTED_EDGE('',*,*,#3566,.T.);
#4419=ORIENTED_EDGE('',*,*,#3569,.F.);
#4420=ORIENTED_EDGE('',*,*,#3570,.T.);
#4421=ORIENTED_EDGE('',*,*,#3571,.T.);
#4422=ORIENTED_EDGE('',*,*,#3570,.F.);
#4423=ORIENTED_EDGE('',*,*,#3571,.F.);
#4424=ORIENTED_EDGE('',*,*,#3572,.F.);
#4425=ORIENTED_EDGE('',*,*,#3573,.T.);
#4426=ORIENTED_EDGE('',*,*,#3574,.T.);
#4427=ORIENTED_EDGE('',*,*,#3573,.F.);
#4428=ORIENTED_EDGE('',*,*,#3574,.F.);
#4429=ORIENTED_EDGE('',*,*,#3575,.F.);
#4430=ORIENTED_EDGE('',*,*,#3576,.T.);
#4431=ORIENTED_EDGE('',*,*,#3577,.T.);
#4432=ORIENTED_EDGE('',*,*,#3576,.F.);
#4433=ORIENTED_EDGE('',*,*,#3577,.F.);
#4434=ORIENTED_EDGE('',*,*,#3578,.F.);
#4435=ORIENTED_EDGE('',*,*,#3579,.T.);
#4436=ORIENTED_EDGE('',*,*,#3580,.T.);
#4437=ORIENTED_EDGE('',*,*,#3579,.F.);
#4438=ORIENTED_EDGE('',*,*,#3580,.F.);
#4439=ORIENTED_EDGE('',*,*,#3581,.F.);
#4440=ORIENTED_EDGE('',*,*,#3582,.F.);
#4441=ORIENTED_EDGE('',*,*,#3583,.F.);
#4442=ORIENTED_EDGE('',*,*,#3584,.F.);
#4443=ORIENTED_EDGE('',*,*,#3585,.F.);
#4444=ORIENTED_EDGE('',*,*,#3586,.F.);
#4445=ORIENTED_EDGE('',*,*,#3587,.F.);
#4446=ORIENTED_EDGE('',*,*,#3588,.F.);
#4447=ORIENTED_EDGE('',*,*,#3589,.F.);
#4448=ORIENTED_EDGE('',*,*,#3584,.T.);
#4449=ORIENTED_EDGE('',*,*,#3590,.F.);
#4450=ORIENTED_EDGE('',*,*,#3586,.T.);
#4451=ORIENTED_EDGE('',*,*,#3591,.F.);
#4452=ORIENTED_EDGE('',*,*,#3592,.F.);
#4453=ORIENTED_EDGE('',*,*,#3593,.F.);
#4454=ORIENTED_EDGE('',*,*,#3594,.F.);
#4455=ORIENTED_EDGE('',*,*,#3595,.F.);
#4456=ORIENTED_EDGE('',*,*,#3596,.F.);
#4457=ORIENTED_EDGE('',*,*,#3597,.F.);
#4458=ORIENTED_EDGE('',*,*,#3598,.F.);
#4459=ORIENTED_EDGE('',*,*,#3599,.F.);
#4460=ORIENTED_EDGE('',*,*,#3600,.F.);
#4461=ORIENTED_EDGE('',*,*,#3595,.T.);
#4462=ORIENTED_EDGE('',*,*,#3601,.F.);
#4463=ORIENTED_EDGE('',*,*,#3597,.T.);
#4464=ORIENTED_EDGE('',*,*,#3602,.F.);
#4465=ORIENTED_EDGE('',*,*,#3603,.F.);
#4466=ORIENTED_EDGE('',*,*,#3604,.F.);
#4467=ORIENTED_EDGE('',*,*,#3605,.F.);
#4468=ORIENTED_EDGE('',*,*,#3606,.F.);
#4469=ORIENTED_EDGE('',*,*,#3607,.F.);
#4470=ORIENTED_EDGE('',*,*,#3608,.F.);
#4471=ORIENTED_EDGE('',*,*,#3609,.F.);
#4472=ORIENTED_EDGE('',*,*,#3610,.F.);
#4473=ORIENTED_EDGE('',*,*,#3611,.F.);
#4474=ORIENTED_EDGE('',*,*,#3606,.T.);
#4475=ORIENTED_EDGE('',*,*,#3612,.F.);
#4476=ORIENTED_EDGE('',*,*,#3608,.T.);
#4477=ORIENTED_EDGE('',*,*,#3613,.F.);
#4478=ORIENTED_EDGE('',*,*,#3614,.F.);
#4479=ORIENTED_EDGE('',*,*,#3615,.F.);
#4480=ORIENTED_EDGE('',*,*,#3616,.F.);
#4481=ORIENTED_EDGE('',*,*,#3617,.F.);
#4482=ORIENTED_EDGE('',*,*,#3618,.F.);
#4483=ORIENTED_EDGE('',*,*,#3619,.F.);
#4484=ORIENTED_EDGE('',*,*,#3620,.F.);
#4485=ORIENTED_EDGE('',*,*,#3621,.F.);
#4486=ORIENTED_EDGE('',*,*,#3622,.F.);
#4487=ORIENTED_EDGE('',*,*,#3617,.T.);
#4488=ORIENTED_EDGE('',*,*,#3623,.F.);
#4489=ORIENTED_EDGE('',*,*,#3619,.T.);
#4490=ORIENTED_EDGE('',*,*,#3624,.F.);
#4491=ORIENTED_EDGE('',*,*,#3582,.T.);
#4492=ORIENTED_EDGE('',*,*,#3625,.F.);
#4493=ORIENTED_EDGE('',*,*,#3626,.T.);
#4494=ORIENTED_EDGE('',*,*,#3627,.F.);
#4495=ORIENTED_EDGE('',*,*,#3588,.T.);
#4496=ORIENTED_EDGE('',*,*,#3628,.F.);
#4497=ORIENTED_EDGE('',*,*,#3629,.F.);
#4498=ORIENTED_EDGE('',*,*,#3630,.F.);
#4499=ORIENTED_EDGE('',*,*,#3593,.T.);
#4500=ORIENTED_EDGE('',*,*,#3631,.F.);
#4501=ORIENTED_EDGE('',*,*,#3632,.F.);
#4502=ORIENTED_EDGE('',*,*,#3633,.F.);
#4503=ORIENTED_EDGE('',*,*,#3599,.T.);
#4504=ORIENTED_EDGE('',*,*,#3634,.F.);
#4505=ORIENTED_EDGE('',*,*,#3635,.F.);
#4506=ORIENTED_EDGE('',*,*,#3636,.F.);
#4507=ORIENTED_EDGE('',*,*,#3587,.T.);
#4508=ORIENTED_EDGE('',*,*,#3590,.T.);
#4509=ORIENTED_EDGE('',*,*,#3583,.T.);
#4510=ORIENTED_EDGE('',*,*,#3627,.T.);
#4511=ORIENTED_EDGE('',*,*,#3637,.T.);
#4512=ORIENTED_EDGE('',*,*,#3638,.T.);
#4513=ORIENTED_EDGE('',*,*,#3639,.T.);
#4514=ORIENTED_EDGE('',*,*,#3640,.T.);
#4515=ORIENTED_EDGE('',*,*,#3609,.T.);
#4516=ORIENTED_EDGE('',*,*,#3612,.T.);
#4517=ORIENTED_EDGE('',*,*,#3605,.T.);
#4518=ORIENTED_EDGE('',*,*,#3641,.T.);
#4519=ORIENTED_EDGE('',*,*,#3642,.F.);
#4520=ORIENTED_EDGE('',*,*,#3628,.T.);
#4521=ORIENTED_EDGE('',*,*,#3604,.T.);
#4522=ORIENTED_EDGE('',*,*,#3643,.F.);
#4523=ORIENTED_EDGE('',*,*,#3644,.F.);
#4524=ORIENTED_EDGE('',*,*,#3641,.F.);
#4525=ORIENTED_EDGE('',*,*,#3610,.T.);
#4526=ORIENTED_EDGE('',*,*,#3640,.F.);
#4527=ORIENTED_EDGE('',*,*,#3645,.F.);
#4528=ORIENTED_EDGE('',*,*,#3646,.F.);
#4529=ORIENTED_EDGE('',*,*,#3598,.T.);
#4530=ORIENTED_EDGE('',*,*,#3601,.T.);
#4531=ORIENTED_EDGE('',*,*,#3594,.T.);
#4532=ORIENTED_EDGE('',*,*,#3633,.T.);
#4533=ORIENTED_EDGE('',*,*,#3647,.F.);
#4534=ORIENTED_EDGE('',*,*,#3648,.T.);
#4535=ORIENTED_EDGE('',*,*,#3620,.T.);
#4536=ORIENTED_EDGE('',*,*,#3623,.T.);
#4537=ORIENTED_EDGE('',*,*,#3616,.T.);
#4538=ORIENTED_EDGE('',*,*,#3649,.T.);
#4539=ORIENTED_EDGE('',*,*,#3650,.T.);
#4540=ORIENTED_EDGE('',*,*,#3651,.T.);
#4541=ORIENTED_EDGE('',*,*,#3652,.T.);
#4542=ORIENTED_EDGE('',*,*,#3634,.T.);
#4543=ORIENTED_EDGE('',*,*,#3615,.T.);
#4544=ORIENTED_EDGE('',*,*,#3653,.F.);
#4545=ORIENTED_EDGE('',*,*,#3654,.T.);
#4546=ORIENTED_EDGE('',*,*,#3649,.F.);
#4547=ORIENTED_EDGE('',*,*,#3621,.T.);
#4548=ORIENTED_EDGE('',*,*,#3648,.F.);
#4549=ORIENTED_EDGE('',*,*,#3655,.F.);
#4550=ORIENTED_EDGE('',*,*,#3656,.F.);
#4551=ORIENTED_EDGE('',*,*,#3657,.F.);
#4552=ORIENTED_EDGE('',*,*,#3658,.T.);
#4553=ORIENTED_EDGE('',*,*,#3591,.T.);
#4554=ORIENTED_EDGE('',*,*,#3658,.F.);
#4555=ORIENTED_EDGE('',*,*,#3659,.F.);
#4556=ORIENTED_EDGE('',*,*,#3660,.T.);
#4557=ORIENTED_EDGE('',*,*,#3602,.T.);
#4558=ORIENTED_EDGE('',*,*,#3660,.F.);
#4559=ORIENTED_EDGE('',*,*,#3661,.F.);
#4560=ORIENTED_EDGE('',*,*,#3662,.T.);
#4561=ORIENTED_EDGE('',*,*,#3613,.T.);
#4562=ORIENTED_EDGE('',*,*,#3662,.F.);
#4563=ORIENTED_EDGE('',*,*,#3663,.F.);
#4564=ORIENTED_EDGE('',*,*,#3664,.T.);
#4565=ORIENTED_EDGE('',*,*,#3624,.T.);
#4566=ORIENTED_EDGE('',*,*,#3664,.F.);
#4567=ORIENTED_EDGE('',*,*,#3665,.F.);
#4568=ORIENTED_EDGE('',*,*,#3635,.T.);
#4569=ORIENTED_EDGE('',*,*,#3652,.F.);
#4570=ORIENTED_EDGE('',*,*,#3666,.F.);
#4571=ORIENTED_EDGE('',*,*,#3667,.F.);
#4572=ORIENTED_EDGE('',*,*,#3666,.T.);
#4573=ORIENTED_EDGE('',*,*,#3651,.F.);
#4574=ORIENTED_EDGE('',*,*,#3668,.F.);
#4575=ORIENTED_EDGE('',*,*,#3659,.T.);
#4576=ORIENTED_EDGE('',*,*,#3663,.T.);
#4577=ORIENTED_EDGE('',*,*,#3669,.F.);
#4578=ORIENTED_EDGE('',*,*,#3668,.T.);
#4579=ORIENTED_EDGE('',*,*,#3650,.F.);
#4580=ORIENTED_EDGE('',*,*,#3654,.F.);
#4581=ORIENTED_EDGE('',*,*,#3596,.T.);
#4582=ORIENTED_EDGE('',*,*,#3636,.T.);
#4583=ORIENTED_EDGE('',*,*,#3665,.T.);
#4584=ORIENTED_EDGE('',*,*,#3667,.T.);
#4585=ORIENTED_EDGE('',*,*,#3669,.T.);
#4586=ORIENTED_EDGE('',*,*,#3653,.T.);
#4587=ORIENTED_EDGE('',*,*,#3614,.T.);
#4588=ORIENTED_EDGE('',*,*,#3622,.T.);
#4589=ORIENTED_EDGE('',*,*,#3618,.T.);
#4590=ORIENTED_EDGE('',*,*,#3656,.T.);
#4591=ORIENTED_EDGE('',*,*,#3670,.F.);
#4592=ORIENTED_EDGE('',*,*,#3631,.T.);
#4593=ORIENTED_EDGE('',*,*,#3592,.T.);
#4594=ORIENTED_EDGE('',*,*,#3600,.T.);
#4595=ORIENTED_EDGE('',*,*,#3671,.F.);
#4596=ORIENTED_EDGE('',*,*,#3645,.T.);
#4597=ORIENTED_EDGE('',*,*,#3639,.F.);
#4598=ORIENTED_EDGE('',*,*,#3672,.F.);
#4599=ORIENTED_EDGE('',*,*,#3673,.F.);
#4600=ORIENTED_EDGE('',*,*,#3672,.T.);
#4601=ORIENTED_EDGE('',*,*,#3638,.F.);
#4602=ORIENTED_EDGE('',*,*,#3674,.F.);
#4603=ORIENTED_EDGE('',*,*,#3657,.T.);
#4604=ORIENTED_EDGE('',*,*,#3661,.T.);
#4605=ORIENTED_EDGE('',*,*,#3675,.F.);
#4606=ORIENTED_EDGE('',*,*,#3674,.T.);
#4607=ORIENTED_EDGE('',*,*,#3637,.F.);
#4608=ORIENTED_EDGE('',*,*,#3626,.F.);
#4609=ORIENTED_EDGE('',*,*,#3585,.T.);
#4610=ORIENTED_EDGE('',*,*,#3630,.T.);
#4611=ORIENTED_EDGE('',*,*,#3676,.F.);
#4612=ORIENTED_EDGE('',*,*,#3643,.T.);
#4613=ORIENTED_EDGE('',*,*,#3603,.T.);
#4614=ORIENTED_EDGE('',*,*,#3611,.T.);
#4615=ORIENTED_EDGE('',*,*,#3607,.T.);
#4616=ORIENTED_EDGE('',*,*,#3646,.T.);
#4617=ORIENTED_EDGE('',*,*,#3671,.T.);
#4618=ORIENTED_EDGE('',*,*,#3673,.T.);
#4619=ORIENTED_EDGE('',*,*,#3675,.T.);
#4620=ORIENTED_EDGE('',*,*,#3625,.T.);
#4621=ORIENTED_EDGE('',*,*,#3581,.T.);
#4622=ORIENTED_EDGE('',*,*,#3589,.T.);
#4623=ORIENTED_EDGE('',*,*,#3677,.F.);
#4624=ORIENTED_EDGE('',*,*,#3678,.T.);
#4625=ORIENTED_EDGE('',*,*,#3679,.T.);
#4626=ORIENTED_EDGE('',*,*,#3678,.F.);
#4627=ORIENTED_EDGE('',*,*,#3680,.F.);
#4628=ORIENTED_EDGE('',*,*,#3681,.T.);
#4629=ORIENTED_EDGE('',*,*,#3682,.T.);
#4630=ORIENTED_EDGE('',*,*,#3681,.F.);
#4631=ORIENTED_EDGE('',*,*,#3655,.T.);
#4632=ORIENTED_EDGE('',*,*,#3647,.T.);
#4633=ORIENTED_EDGE('',*,*,#3632,.T.);
#4634=ORIENTED_EDGE('',*,*,#3670,.T.);
#4635=ORIENTED_EDGE('',*,*,#3629,.T.);
#4636=ORIENTED_EDGE('',*,*,#3642,.T.);
#4637=ORIENTED_EDGE('',*,*,#3644,.T.);
#4638=ORIENTED_EDGE('',*,*,#3676,.T.);
#4639=ORIENTED_EDGE('',*,*,#3680,.T.);
#4640=ORIENTED_EDGE('',*,*,#3677,.T.);
#4641=ORIENTED_EDGE('',*,*,#3568,.T.);
#4642=ORIENTED_EDGE('',*,*,#3565,.T.);
#4643=ORIENTED_EDGE('',*,*,#3562,.T.);
#4644=ORIENTED_EDGE('',*,*,#3559,.T.);
#4645=ORIENTED_EDGE('',*,*,#3682,.F.);
#4646=ORIENTED_EDGE('',*,*,#3679,.F.);
#4647=ORIENTED_EDGE('',*,*,#3578,.T.);
#4648=ORIENTED_EDGE('',*,*,#3575,.T.);
#4649=ORIENTED_EDGE('',*,*,#3572,.T.);
#4650=ORIENTED_EDGE('',*,*,#3569,.T.);
#5991=CYLINDRICAL_SURFACE('',#6982,0.165);
#5992=CYLINDRICAL_SURFACE('',#6986,0.165);
#5993=CYLINDRICAL_SURFACE('',#6990,0.165);
#5994=CYLINDRICAL_SURFACE('',#6994,0.165);
#5995=CYLINDRICAL_SURFACE('',#6998,0.165);
#5996=CYLINDRICAL_SURFACE('',#7002,0.165);
#5997=CYLINDRICAL_SURFACE('',#7006,0.165);
#5998=CYLINDRICAL_SURFACE('',#7010,0.165);
#5999=CYLINDRICAL_SURFACE('',#7014,0.6);
#6000=CYLINDRICAL_SURFACE('',#7017,0.6);
#6001=CYLINDRICAL_SURFACE('',#7022,0.6);
#6002=CYLINDRICAL_SURFACE('',#7025,0.6);
#6003=CYLINDRICAL_SURFACE('',#7030,0.6);
#6004=CYLINDRICAL_SURFACE('',#7033,0.6);
#6005=CYLINDRICAL_SURFACE('',#7038,0.6);
#6006=CYLINDRICAL_SURFACE('',#7041,0.6);
#6007=CYLINDRICAL_SURFACE('',#7058,0.33);
#6008=CYLINDRICAL_SURFACE('',#7060,0.33);
#6009=CYLINDRICAL_SURFACE('',#7062,0.33);
#6010=CYLINDRICAL_SURFACE('',#7064,0.33);
#6011=CYLINDRICAL_SURFACE('',#7076,2.6);
#6012=CYLINDRICAL_SURFACE('',#7079,4.);
#6110=ADVANCED_FACE('',(#885),#5991,.F.);
#6111=ADVANCED_FACE('',(#886),#658,.T.);
#6112=ADVANCED_FACE('',(#887),#5992,.F.);
#6113=ADVANCED_FACE('',(#888),#659,.T.);
#6114=ADVANCED_FACE('',(#889),#5993,.F.);
#6115=ADVANCED_FACE('',(#890),#660,.T.);
#6116=ADVANCED_FACE('',(#891),#5994,.F.);
#6117=ADVANCED_FACE('',(#892),#661,.T.);
#6118=ADVANCED_FACE('',(#893),#5995,.F.);
#6119=ADVANCED_FACE('',(#894),#662,.F.);
#6120=ADVANCED_FACE('',(#895),#5996,.F.);
#6121=ADVANCED_FACE('',(#896),#663,.F.);
#6122=ADVANCED_FACE('',(#897),#5997,.F.);
#6123=ADVANCED_FACE('',(#898),#664,.F.);
#6124=ADVANCED_FACE('',(#899),#5998,.F.);
#6125=ADVANCED_FACE('',(#900),#665,.F.);
#6126=ADVANCED_FACE('',(#901),#5999,.F.);
#6127=ADVANCED_FACE('',(#902),#6000,.F.);
#6128=ADVANCED_FACE('',(#903,#539),#666,.T.);
#6129=ADVANCED_FACE('',(#904),#6001,.F.);
#6130=ADVANCED_FACE('',(#905),#6002,.F.);
#6131=ADVANCED_FACE('',(#906,#540),#667,.T.);
#6132=ADVANCED_FACE('',(#907),#6003,.F.);
#6133=ADVANCED_FACE('',(#908),#6004,.F.);
#6134=ADVANCED_FACE('',(#909,#541),#668,.T.);
#6135=ADVANCED_FACE('',(#910),#6005,.F.);
#6136=ADVANCED_FACE('',(#911),#6006,.F.);
#6137=ADVANCED_FACE('',(#912,#542),#669,.T.);
#6138=ADVANCED_FACE('',(#913),#670,.T.);
#6139=ADVANCED_FACE('',(#914),#671,.T.);
#6140=ADVANCED_FACE('',(#915),#672,.T.);
#6141=ADVANCED_FACE('',(#916),#673,.T.);
#6142=ADVANCED_FACE('',(#917),#674,.T.);
#6143=ADVANCED_FACE('',(#918),#675,.T.);
#6144=ADVANCED_FACE('',(#919),#676,.T.);
#6145=ADVANCED_FACE('',(#920),#677,.T.);
#6146=ADVANCED_FACE('',(#921),#678,.T.);
#6147=ADVANCED_FACE('',(#922),#679,.T.);
#6148=ADVANCED_FACE('',(#923),#6007,.F.);
#6149=ADVANCED_FACE('',(#924),#6008,.F.);
#6150=ADVANCED_FACE('',(#925),#6009,.F.);
#6151=ADVANCED_FACE('',(#926),#6010,.F.);
#6152=ADVANCED_FACE('',(#927),#680,.T.);
#6153=ADVANCED_FACE('',(#928,#543,#544),#681,.T.);
#6154=ADVANCED_FACE('',(#929),#682,.T.);
#6155=ADVANCED_FACE('',(#930),#683,.F.);
#6156=ADVANCED_FACE('',(#931),#684,.T.);
#6157=ADVANCED_FACE('',(#932,#545,#546),#685,.T.);
#6158=ADVANCED_FACE('',(#933),#686,.T.);
#6159=ADVANCED_FACE('',(#934),#687,.F.);
#6160=ADVANCED_FACE('',(#935),#6011,.F.);
#6161=ADVANCED_FACE('',(#936,#547,#548),#6012,.T.);
#6162=ADVANCED_FACE('',(#937,#549,#550,#551,#552,#553),#688,.T.);
#6163=ADVANCED_FACE('',(#938,#554,#555,#556,#557,#558),#689,.F.);
#6496=CLOSED_SHELL('',(#6110,#6111,#6112,#6113,#6114,#6115,#6116,#6117,
#6118,#6119,#6120,#6121,#6122,#6123,#6124,#6125,#6126,#6127,#6128,#6129,
#6130,#6131,#6132,#6133,#6134,#6135,#6136,#6137,#6138,#6139,#6140,#6141,
#6142,#6143,#6144,#6145,#6146,#6147,#6148,#6149,#6150,#6151,#6152,#6153,
#6154,#6155,#6156,#6157,#6158,#6159,#6160,#6161,#6162,#6163));
#6981=AXIS2_PLACEMENT_3D('',#9978,#7868,#7869);
#6982=AXIS2_PLACEMENT_3D('',#9979,#7870,#7871);
#6983=AXIS2_PLACEMENT_3D('',#9981,#7872,#7873);
#6984=AXIS2_PLACEMENT_3D('',#9984,#7875,#7876);
#6985=AXIS2_PLACEMENT_3D('',#9985,#7877,#7878);
#6986=AXIS2_PLACEMENT_3D('',#9986,#7879,#7880);
#6987=AXIS2_PLACEMENT_3D('',#9988,#7881,#7882);
#6988=AXIS2_PLACEMENT_3D('',#9991,#7884,#7885);
#6989=AXIS2_PLACEMENT_3D('',#9992,#7886,#7887);
#6990=AXIS2_PLACEMENT_3D('',#9993,#7888,#7889);
#6991=AXIS2_PLACEMENT_3D('',#9995,#7890,#7891);
#6992=AXIS2_PLACEMENT_3D('',#9998,#7893,#7894);
#6993=AXIS2_PLACEMENT_3D('',#9999,#7895,#7896);
#6994=AXIS2_PLACEMENT_3D('',#10000,#7897,#7898);
#6995=AXIS2_PLACEMENT_3D('',#10002,#7899,#7900);
#6996=AXIS2_PLACEMENT_3D('',#10005,#7902,#7903);
#6997=AXIS2_PLACEMENT_3D('',#10006,#7904,#7905);
#6998=AXIS2_PLACEMENT_3D('',#10007,#7906,#7907);
#6999=AXIS2_PLACEMENT_3D('',#10009,#7908,#7909);
#7000=AXIS2_PLACEMENT_3D('',#10012,#7911,#7912);
#7001=AXIS2_PLACEMENT_3D('',#10013,#7913,#7914);
#7002=AXIS2_PLACEMENT_3D('',#10014,#7915,#7916);
#7003=AXIS2_PLACEMENT_3D('',#10016,#7917,#7918);
#7004=AXIS2_PLACEMENT_3D('',#10019,#7920,#7921);
#7005=AXIS2_PLACEMENT_3D('',#10020,#7922,#7923);
#7006=AXIS2_PLACEMENT_3D('',#10021,#7924,#7925);
#7007=AXIS2_PLACEMENT_3D('',#10023,#7926,#7927);
#7008=AXIS2_PLACEMENT_3D('',#10026,#7929,#7930);
#7009=AXIS2_PLACEMENT_3D('',#10027,#7931,#7932);
#7010=AXIS2_PLACEMENT_3D('',#10028,#7933,#7934);
#7011=AXIS2_PLACEMENT_3D('',#10030,#7935,#7936);
#7012=AXIS2_PLACEMENT_3D('',#10033,#7938,#7939);
#7013=AXIS2_PLACEMENT_3D('',#10034,#7940,#7941);
#7014=AXIS2_PLACEMENT_3D('',#10035,#7942,#7943);
#7015=AXIS2_PLACEMENT_3D('',#10040,#7945,#7946);
#7016=AXIS2_PLACEMENT_3D('',#10043,#7948,#7949);
#7017=AXIS2_PLACEMENT_3D('',#10044,#7950,#7951);
#7018=AXIS2_PLACEMENT_3D('',#10049,#7953,#7954);
#7019=AXIS2_PLACEMENT_3D('',#10052,#7956,#7957);
#7020=AXIS2_PLACEMENT_3D('',#10053,#7958,#7959);
#7021=AXIS2_PLACEMENT_3D('',#10057,#7962,#7963);
#7022=AXIS2_PLACEMENT_3D('',#10058,#7964,#7965);
#7023=AXIS2_PLACEMENT_3D('',#10063,#7967,#7968);
#7024=AXIS2_PLACEMENT_3D('',#10066,#7970,#7971);
#7025=AXIS2_PLACEMENT_3D('',#10067,#7972,#7973);
#7026=AXIS2_PLACEMENT_3D('',#10072,#7975,#7976);
#7027=AXIS2_PLACEMENT_3D('',#10075,#7978,#7979);
#7028=AXIS2_PLACEMENT_3D('',#10076,#7980,#7981);
#7029=AXIS2_PLACEMENT_3D('',#10080,#7984,#7985);
#7030=AXIS2_PLACEMENT_3D('',#10081,#7986,#7987);
#7031=AXIS2_PLACEMENT_3D('',#10086,#7989,#7990);
#7032=AXIS2_PLACEMENT_3D('',#10089,#7992,#7993);
#7033=AXIS2_PLACEMENT_3D('',#10090,#7994,#7995);
#7034=AXIS2_PLACEMENT_3D('',#10095,#7997,#7998);
#7035=AXIS2_PLACEMENT_3D('',#10098,#8000,#8001);
#7036=AXIS2_PLACEMENT_3D('',#10099,#8002,#8003);
#7037=AXIS2_PLACEMENT_3D('',#10103,#8006,#8007);
#7038=AXIS2_PLACEMENT_3D('',#10104,#8008,#8009);
#7039=AXIS2_PLACEMENT_3D('',#10109,#8011,#8012);
#7040=AXIS2_PLACEMENT_3D('',#10112,#8014,#8015);
#7041=AXIS2_PLACEMENT_3D('',#10113,#8016,#8017);
#7042=AXIS2_PLACEMENT_3D('',#10118,#8019,#8020);
#7043=AXIS2_PLACEMENT_3D('',#10121,#8022,#8023);
#7044=AXIS2_PLACEMENT_3D('',#10122,#8024,#8025);
#7045=AXIS2_PLACEMENT_3D('',#10126,#8028,#8029);
#7046=AXIS2_PLACEMENT_3D('',#10127,#8030,#8031);
#7047=AXIS2_PLACEMENT_3D('',#10133,#8035,#8036);
#7048=AXIS2_PLACEMENT_3D('',#10139,#8040,#8041);
#7049=AXIS2_PLACEMENT_3D('',#10145,#8045,#8046);
#7050=AXIS2_PLACEMENT_3D('',#10151,#8050,#8051);
#7051=AXIS2_PLACEMENT_3D('',#10161,#8057,#8058);
#7052=AXIS2_PLACEMENT_3D('',#10162,#8059,#8060);
#7053=AXIS2_PLACEMENT_3D('',#10166,#8063,#8064);
#7054=AXIS2_PLACEMENT_3D('',#10170,#8067,#8068);
#7055=AXIS2_PLACEMENT_3D('',#10172,#8069,#8070);
#7056=AXIS2_PLACEMENT_3D('',#10181,#8076,#8077);
#7057=AXIS2_PLACEMENT_3D('',#10185,#8080,#8081);
#7058=AXIS2_PLACEMENT_3D('',#10189,#8084,#8085);
#7059=AXIS2_PLACEMENT_3D('',#10191,#8086,#8087);
#7060=AXIS2_PLACEMENT_3D('',#10193,#8089,#8090);
#7061=AXIS2_PLACEMENT_3D('',#10195,#8091,#8092);
#7062=AXIS2_PLACEMENT_3D('',#10197,#8094,#8095);
#7063=AXIS2_PLACEMENT_3D('',#10199,#8096,#8097);
#7064=AXIS2_PLACEMENT_3D('',#10201,#8099,#8100);
#7065=AXIS2_PLACEMENT_3D('',#10203,#8101,#8102);
#7066=AXIS2_PLACEMENT_3D('',#10205,#8104,#8105);
#7067=AXIS2_PLACEMENT_3D('',#10209,#8108,#8109);
#7068=AXIS2_PLACEMENT_3D('',#10213,#8112,#8113);
#7069=AXIS2_PLACEMENT_3D('',#10215,#8115,#8116);
#7070=AXIS2_PLACEMENT_3D('',#10216,#8117,#8118);
#7071=AXIS2_PLACEMENT_3D('',#10217,#8119,#8120);
#7072=AXIS2_PLACEMENT_3D('',#10221,#8123,#8124);
#7073=AXIS2_PLACEMENT_3D('',#10225,#8127,#8128);
#7074=AXIS2_PLACEMENT_3D('',#10227,#8130,#8131);
#7075=AXIS2_PLACEMENT_3D('',#10228,#8132,#8133);
#7076=AXIS2_PLACEMENT_3D('',#10229,#8134,#8135);
#7077=AXIS2_PLACEMENT_3D('',#10231,#8136,#8137);
#7078=AXIS2_PLACEMENT_3D('',#10234,#8139,#8140);
#7079=AXIS2_PLACEMENT_3D('',#10235,#8141,#8142);
#7080=AXIS2_PLACEMENT_3D('',#10237,#8143,#8144);
#7081=AXIS2_PLACEMENT_3D('',#10240,#8146,#8147);
#7082=AXIS2_PLACEMENT_3D('',#10241,#8148,#8149);
#7083=AXIS2_PLACEMENT_3D('',#10242,#8150,#8151);
#7868=DIRECTION('axis',(0.,0.,1.));
#7869=DIRECTION('refdir',(1.,0.,0.));
#7870=DIRECTION('center_axis',(0.,1.,0.));
#7871=DIRECTION('ref_axis',(1.,0.,0.));
#7872=DIRECTION('center_axis',(0.,1.,0.));
#7873=DIRECTION('ref_axis',(1.,0.,0.));
#7874=DIRECTION('',(0.,1.,0.));
#7875=DIRECTION('center_axis',(0.,-1.,0.));
#7876=DIRECTION('ref_axis',(1.,0.,0.));
#7877=DIRECTION('center_axis',(0.,1.,0.));
#7878=DIRECTION('ref_axis',(1.,0.,0.));
#7879=DIRECTION('center_axis',(0.,1.,0.));
#7880=DIRECTION('ref_axis',(1.,0.,0.));
#7881=DIRECTION('center_axis',(0.,1.,0.));
#7882=DIRECTION('ref_axis',(1.,0.,0.));
#7883=DIRECTION('',(0.,1.,0.));
#7884=DIRECTION('center_axis',(0.,-1.,0.));
#7885=DIRECTION('ref_axis',(1.,0.,0.));
#7886=DIRECTION('center_axis',(0.,1.,0.));
#7887=DIRECTION('ref_axis',(1.,0.,0.));
#7888=DIRECTION('center_axis',(0.,1.,0.));
#7889=DIRECTION('ref_axis',(1.,0.,0.));
#7890=DIRECTION('center_axis',(0.,1.,0.));
#7891=DIRECTION('ref_axis',(1.,0.,0.));
#7892=DIRECTION('',(0.,1.,0.));
#7893=DIRECTION('center_axis',(0.,-1.,0.));
#7894=DIRECTION('ref_axis',(1.,0.,0.));
#7895=DIRECTION('center_axis',(0.,1.,0.));
#7896=DIRECTION('ref_axis',(1.,0.,0.));
#7897=DIRECTION('center_axis',(0.,1.,0.));
#7898=DIRECTION('ref_axis',(1.,0.,0.));
#7899=DIRECTION('center_axis',(0.,1.,0.));
#7900=DIRECTION('ref_axis',(1.,0.,0.));
#7901=DIRECTION('',(0.,1.,0.));
#7902=DIRECTION('center_axis',(0.,-1.,0.));
#7903=DIRECTION('ref_axis',(1.,0.,0.));
#7904=DIRECTION('center_axis',(0.,1.,0.));
#7905=DIRECTION('ref_axis',(1.,0.,0.));
#7906=DIRECTION('center_axis',(0.,1.,0.));
#7907=DIRECTION('ref_axis',(1.,0.,0.));
#7908=DIRECTION('center_axis',(0.,1.,0.));
#7909=DIRECTION('ref_axis',(1.,0.,0.));
#7910=DIRECTION('',(0.,1.,0.));
#7911=DIRECTION('center_axis',(0.,1.,0.));
#7912=DIRECTION('ref_axis',(1.,0.,0.));
#7913=DIRECTION('center_axis',(0.,1.,0.));
#7914=DIRECTION('ref_axis',(1.,0.,0.));
#7915=DIRECTION('center_axis',(0.,1.,0.));
#7916=DIRECTION('ref_axis',(1.,0.,0.));
#7917=DIRECTION('center_axis',(0.,1.,0.));
#7918=DIRECTION('ref_axis',(1.,0.,0.));
#7919=DIRECTION('',(0.,1.,0.));
#7920=DIRECTION('center_axis',(0.,1.,0.));
#7921=DIRECTION('ref_axis',(1.,0.,0.));
#7922=DIRECTION('center_axis',(0.,1.,0.));
#7923=DIRECTION('ref_axis',(1.,0.,0.));
#7924=DIRECTION('center_axis',(0.,1.,0.));
#7925=DIRECTION('ref_axis',(1.,0.,0.));
#7926=DIRECTION('center_axis',(0.,1.,0.));
#7927=DIRECTION('ref_axis',(1.,0.,0.));
#7928=DIRECTION('',(0.,1.,0.));
#7929=DIRECTION('center_axis',(0.,1.,0.));
#7930=DIRECTION('ref_axis',(1.,0.,0.));
#7931=DIRECTION('center_axis',(0.,1.,0.));
#7932=DIRECTION('ref_axis',(1.,0.,0.));
#7933=DIRECTION('center_axis',(0.,1.,0.));
#7934=DIRECTION('ref_axis',(1.,0.,0.));
#7935=DIRECTION('center_axis',(0.,1.,0.));
#7936=DIRECTION('ref_axis',(1.,0.,0.));
#7937=DIRECTION('',(0.,1.,0.));
#7938=DIRECTION('center_axis',(0.,1.,0.));
#7939=DIRECTION('ref_axis',(1.,0.,0.));
#7940=DIRECTION('center_axis',(0.,1.,0.));
#7941=DIRECTION('ref_axis',(1.,0.,0.));
#7942=DIRECTION('center_axis',(0.,0.,1.));
#7943=DIRECTION('ref_axis',(1.,0.,0.));
#7944=DIRECTION('',(0.,0.,-1.));
#7945=DIRECTION('center_axis',(0.,0.,-1.));
#7946=DIRECTION('ref_axis',(1.,0.,0.));
#7947=DIRECTION('',(0.,0.,1.));
#7948=DIRECTION('center_axis',(0.,0.,1.));
#7949=DIRECTION('ref_axis',(1.,0.,0.));
#7950=DIRECTION('center_axis',(0.,0.,1.));
#7951=DIRECTION('ref_axis',(-1.,-1.22464679914735E-16,0.));
#7952=DIRECTION('',(0.,0.,1.));
#7953=DIRECTION('center_axis',(0.,0.,1.));
#7954=DIRECTION('ref_axis',(1.,0.,0.));
#7955=DIRECTION('',(0.,0.,-1.));
#7956=DIRECTION('center_axis',(0.,0.,-1.));
#7957=DIRECTION('ref_axis',(1.,0.,0.));
#7958=DIRECTION('center_axis',(0.,0.,1.));
#7959=DIRECTION('ref_axis',(1.,0.,0.));
#7960=DIRECTION('',(-1.,0.,0.));
#7961=DIRECTION('',(1.,0.,0.));
#7962=DIRECTION('center_axis',(0.,0.,1.));
#7963=DIRECTION('ref_axis',(1.,0.,0.));
#7964=DIRECTION('center_axis',(0.,0.,1.));
#7965=DIRECTION('ref_axis',(1.,0.,0.));
#7966=DIRECTION('',(0.,0.,-1.));
#7967=DIRECTION('center_axis',(0.,0.,-1.));
#7968=DIRECTION('ref_axis',(1.,0.,0.));
#7969=DIRECTION('',(0.,0.,1.));
#7970=DIRECTION('center_axis',(0.,0.,1.));
#7971=DIRECTION('ref_axis',(1.,0.,0.));
#7972=DIRECTION('center_axis',(0.,0.,1.));
#7973=DIRECTION('ref_axis',(-1.,-1.22464679914735E-16,0.));
#7974=DIRECTION('',(0.,0.,1.));
#7975=DIRECTION('center_axis',(0.,0.,1.));
#7976=DIRECTION('ref_axis',(1.,0.,0.));
#7977=DIRECTION('',(0.,0.,-1.));
#7978=DIRECTION('center_axis',(0.,0.,-1.));
#7979=DIRECTION('ref_axis',(1.,0.,0.));
#7980=DIRECTION('center_axis',(0.,0.,1.));
#7981=DIRECTION('ref_axis',(1.,0.,0.));
#7982=DIRECTION('',(-1.,0.,0.));
#7983=DIRECTION('',(1.,0.,0.));
#7984=DIRECTION('center_axis',(0.,0.,1.));
#7985=DIRECTION('ref_axis',(1.,0.,0.));
#7986=DIRECTION('center_axis',(0.,0.,1.));
#7987=DIRECTION('ref_axis',(1.,0.,0.));
#7988=DIRECTION('',(0.,0.,-1.));
#7989=DIRECTION('center_axis',(0.,0.,-1.));
#7990=DIRECTION('ref_axis',(1.,0.,0.));
#7991=DIRECTION('',(0.,0.,1.));
#7992=DIRECTION('center_axis',(0.,0.,1.));
#7993=DIRECTION('ref_axis',(1.,0.,0.));
#7994=DIRECTION('center_axis',(0.,0.,1.));
#7995=DIRECTION('ref_axis',(-1.,-1.22464679914735E-16,0.));
#7996=DIRECTION('',(0.,0.,1.));
#7997=DIRECTION('center_axis',(0.,0.,1.));
#7998=DIRECTION('ref_axis',(1.,0.,0.));
#7999=DIRECTION('',(0.,0.,-1.));
#8000=DIRECTION('center_axis',(0.,0.,-1.));
#8001=DIRECTION('ref_axis',(1.,0.,0.));
#8002=DIRECTION('center_axis',(0.,0.,1.));
#8003=DIRECTION('ref_axis',(1.,0.,0.));
#8004=DIRECTION('',(-1.,0.,0.));
#8005=DIRECTION('',(1.,0.,0.));
#8006=DIRECTION('center_axis',(0.,0.,1.));
#8007=DIRECTION('ref_axis',(1.,0.,0.));
#8008=DIRECTION('center_axis',(0.,0.,1.));
#8009=DIRECTION('ref_axis',(1.,0.,0.));
#8010=DIRECTION('',(0.,0.,-1.));
#8011=DIRECTION('center_axis',(0.,0.,-1.));
#8012=DIRECTION('ref_axis',(1.,0.,0.));
#8013=DIRECTION('',(0.,0.,1.));
#8014=DIRECTION('center_axis',(0.,0.,1.));
#8015=DIRECTION('ref_axis',(1.,0.,0.));
#8016=DIRECTION('center_axis',(0.,0.,1.));
#8017=DIRECTION('ref_axis',(-1.,-1.22464679914735E-16,0.));
#8018=DIRECTION('',(0.,0.,1.));
#8019=DIRECTION('center_axis',(0.,0.,1.));
#8020=DIRECTION('ref_axis',(1.,0.,0.));
#8021=DIRECTION('',(0.,0.,-1.));
#8022=DIRECTION('center_axis',(0.,0.,-1.));
#8023=DIRECTION('ref_axis',(1.,0.,0.));
#8024=DIRECTION('center_axis',(0.,0.,1.));
#8025=DIRECTION('ref_axis',(1.,0.,0.));
#8026=DIRECTION('',(-1.,0.,0.));
#8027=DIRECTION('',(1.,0.,0.));
#8028=DIRECTION('center_axis',(0.,0.,1.));
#8029=DIRECTION('ref_axis',(1.,0.,0.));
#8030=DIRECTION('center_axis',(0.,0.,1.));
#8031=DIRECTION('ref_axis',(1.,0.,0.));
#8032=DIRECTION('',(-1.,0.,0.));
#8033=DIRECTION('',(0.,1.,0.));
#8034=DIRECTION('',(1.,0.,0.));
#8035=DIRECTION('center_axis',(0.,0.,1.));
#8036=DIRECTION('ref_axis',(1.,0.,0.));
#8037=DIRECTION('',(1.,0.,0.));
#8038=DIRECTION('',(0.,1.,0.));
#8039=DIRECTION('',(-1.,0.,0.));
#8040=DIRECTION('center_axis',(0.,0.,1.));
#8041=DIRECTION('ref_axis',(1.,0.,0.));
#8042=DIRECTION('',(-1.,0.,0.));
#8043=DIRECTION('',(0.,-1.,0.));
#8044=DIRECTION('',(1.,0.,0.));
#8045=DIRECTION('center_axis',(0.,0.,1.));
#8046=DIRECTION('ref_axis',(1.,0.,0.));
#8047=DIRECTION('',(1.,0.,0.));
#8048=DIRECTION('',(0.,1.,0.));
#8049=DIRECTION('',(-1.,0.,0.));
#8050=DIRECTION('center_axis',(0.,1.,0.));
#8051=DIRECTION('ref_axis',(0.,0.,1.));
#8052=DIRECTION('',(0.,0.,-1.));
#8053=DIRECTION('',(-1.,0.,0.));
#8054=DIRECTION('',(0.,0.,1.));
#8055=DIRECTION('',(1.,0.,0.));
#8056=DIRECTION('',(1.,0.,0.));
#8057=DIRECTION('center_axis',(0.,1.,0.));
#8058=DIRECTION('ref_axis',(1.,0.,0.));
#8059=DIRECTION('center_axis',(0.,0.,1.));
#8060=DIRECTION('ref_axis',(1.,0.,0.));
#8061=DIRECTION('',(-1.,0.,0.));
#8062=DIRECTION('',(0.,-1.,0.));
#8063=DIRECTION('center_axis',(0.,0.,1.));
#8064=DIRECTION('ref_axis',(1.,0.,0.));
#8065=DIRECTION('',(0.,1.,0.));
#8066=DIRECTION('',(-1.,0.,0.));
#8067=DIRECTION('center_axis',(0.,1.,0.));
#8068=DIRECTION('ref_axis',(0.,0.,1.));
#8069=DIRECTION('center_axis',(0.,1.,0.));
#8070=DIRECTION('ref_axis',(1.,0.,0.));
#8071=DIRECTION('',(1.,0.,0.));
#8072=DIRECTION('',(1.,0.,0.));
#8073=DIRECTION('',(0.,0.,-1.));
#8074=DIRECTION('',(-1.,0.,0.));
#8075=DIRECTION('',(0.,0.,1.));
#8076=DIRECTION('center_axis',(0.,0.,1.));
#8077=DIRECTION('ref_axis',(1.,0.,0.));
#8078=DIRECTION('',(-1.,0.,0.));
#8079=DIRECTION('',(0.,1.,0.));
#8080=DIRECTION('center_axis',(0.,0.,1.));
#8081=DIRECTION('ref_axis',(1.,0.,0.));
#8082=DIRECTION('',(0.,1.,0.));
#8083=DIRECTION('',(-1.,0.,0.));
#8084=DIRECTION('center_axis',(0.,0.,1.));
#8085=DIRECTION('ref_axis',(1.,0.,0.));
#8086=DIRECTION('center_axis',(0.,0.,1.));
#8087=DIRECTION('ref_axis',(1.,0.,0.));
#8088=DIRECTION('',(0.,0.,1.));
#8089=DIRECTION('center_axis',(0.,0.,1.));
#8090=DIRECTION('ref_axis',(1.,0.,0.));
#8091=DIRECTION('center_axis',(0.,0.,1.));
#8092=DIRECTION('ref_axis',(1.,0.,0.));
#8093=DIRECTION('',(0.,0.,1.));
#8094=DIRECTION('center_axis',(0.,0.,1.));
#8095=DIRECTION('ref_axis',(1.,0.,0.));
#8096=DIRECTION('center_axis',(0.,0.,1.));
#8097=DIRECTION('ref_axis',(1.,0.,0.));
#8098=DIRECTION('',(0.,0.,1.));
#8099=DIRECTION('center_axis',(0.,0.,1.));
#8100=DIRECTION('ref_axis',(1.,0.,0.));
#8101=DIRECTION('center_axis',(0.,0.,1.));
#8102=DIRECTION('ref_axis',(1.,0.,0.));
#8103=DIRECTION('',(0.,0.,1.));
#8104=DIRECTION('center_axis',(-1.,0.,0.));
#8105=DIRECTION('ref_axis',(0.,0.,1.));
#8106=DIRECTION('',(0.,0.,-1.));
#8107=DIRECTION('',(0.,1.,0.));
#8108=DIRECTION('center_axis',(0.,0.,-1.));
#8109=DIRECTION('ref_axis',(-1.,0.,0.));
#8110=DIRECTION('',(1.,0.,0.));
#8111=DIRECTION('',(0.,1.,0.));
#8112=DIRECTION('center_axis',(1.,0.,0.));
#8113=DIRECTION('ref_axis',(0.,0.,-1.));
#8114=DIRECTION('',(0.,0.,1.));
#8115=DIRECTION('center_axis',(0.,1.,0.));
#8116=DIRECTION('ref_axis',(1.,0.,0.));
#8117=DIRECTION('center_axis',(0.,-1.,0.));
#8118=DIRECTION('ref_axis',(1.,0.,0.));
#8119=DIRECTION('center_axis',(-1.,0.,0.));
#8120=DIRECTION('ref_axis',(0.,0.,1.));
#8121=DIRECTION('',(0.,0.,-1.));
#8122=DIRECTION('',(0.,1.,0.));
#8123=DIRECTION('center_axis',(0.,0.,-1.));
#8124=DIRECTION('ref_axis',(-1.,0.,0.));
#8125=DIRECTION('',(1.,0.,0.));
#8126=DIRECTION('',(0.,1.,0.));
#8127=DIRECTION('center_axis',(1.,0.,0.));
#8128=DIRECTION('ref_axis',(0.,0.,-1.));
#8129=DIRECTION('',(0.,0.,1.));
#8130=DIRECTION('center_axis',(0.,1.,0.));
#8131=DIRECTION('ref_axis',(1.,0.,0.));
#8132=DIRECTION('center_axis',(0.,-1.,0.));
#8133=DIRECTION('ref_axis',(1.,0.,0.));
#8134=DIRECTION('center_axis',(0.,1.,0.));
#8135=DIRECTION('ref_axis',(1.,0.,0.));
#8136=DIRECTION('center_axis',(0.,-1.,0.));
#8137=DIRECTION('ref_axis',(1.,0.,0.));
#8138=DIRECTION('',(0.,-1.,0.));
#8139=DIRECTION('center_axis',(0.,-1.,0.));
#8140=DIRECTION('ref_axis',(1.,0.,0.));
#8141=DIRECTION('center_axis',(0.,1.,0.));
#8142=DIRECTION('ref_axis',(1.,0.,0.));
#8143=DIRECTION('center_axis',(0.,1.,0.));
#8144=DIRECTION('ref_axis',(1.,0.,0.));
#8145=DIRECTION('',(0.,-1.,0.));
#8146=DIRECTION('center_axis',(0.,1.,0.));
#8147=DIRECTION('ref_axis',(1.,0.,0.));
#8148=DIRECTION('center_axis',(0.,1.,0.));
#8149=DIRECTION('ref_axis',(1.,0.,0.));
#8150=DIRECTION('center_axis',(0.,1.,0.));
#8151=DIRECTION('ref_axis',(1.,0.,0.));
#9978=CARTESIAN_POINT('',(0.,0.,0.));
#9979=CARTESIAN_POINT('Origin',(-3.3,4.4,8.));
#9980=CARTESIAN_POINT('',(-3.465,4.4,8.));
#9981=CARTESIAN_POINT('Origin',(-3.3,4.4,8.));
#9982=CARTESIAN_POINT('',(-3.465,6.,8.));
#9983=CARTESIAN_POINT('',(-3.465,4.4,8.));
#9984=CARTESIAN_POINT('Origin',(-3.3,6.,8.));
#9985=CARTESIAN_POINT('Origin',(-3.3,4.4,8.));
#9986=CARTESIAN_POINT('Origin',(2.02066721859313E-16,4.4,11.3));
#9987=CARTESIAN_POINT('',(-0.165,4.4,11.3));
#9988=CARTESIAN_POINT('Origin',(2.02066721859313E-16,4.4,11.3));
#9989=CARTESIAN_POINT('',(-0.165,6.,11.3));
#9990=CARTESIAN_POINT('',(-0.165,4.4,11.3));
#9991=CARTESIAN_POINT('Origin',(2.02066721859313E-16,6.,11.3));
#9992=CARTESIAN_POINT('Origin',(1.94289029309402E-16,4.4,11.3));
#9993=CARTESIAN_POINT('Origin',(3.3,4.4,8.));
#9994=CARTESIAN_POINT('',(3.135,4.4,8.));
#9995=CARTESIAN_POINT('Origin',(3.3,4.4,8.));
#9996=CARTESIAN_POINT('',(3.135,6.,8.));
#9997=CARTESIAN_POINT('',(3.135,4.4,8.));
#9998=CARTESIAN_POINT('Origin',(3.3,6.,8.));
#9999=CARTESIAN_POINT('Origin',(3.3,4.4,8.));
#10000=CARTESIAN_POINT('Origin',(-6.0620016557794E-16,4.4,4.7));
#10001=CARTESIAN_POINT('',(-0.165000000000001,4.4,4.7));
#10002=CARTESIAN_POINT('Origin',(-6.0620016557794E-16,4.4,4.7));
#10003=CARTESIAN_POINT('',(-0.165000000000001,6.,4.7));
#10004=CARTESIAN_POINT('',(-0.165000000000001,4.4,4.7));
#10005=CARTESIAN_POINT('Origin',(-6.0620016557794E-16,6.,4.7));
#10006=CARTESIAN_POINT('Origin',(-6.10622663543836E-16,4.4,4.7));
#10007=CARTESIAN_POINT('Origin',(-3.3,-0.1,8.));
#10008=CARTESIAN_POINT('',(-3.465,0.,8.));
#10009=CARTESIAN_POINT('Origin',(-3.3,0.,8.));
#10010=CARTESIAN_POINT('',(-3.465,1.6,8.));
#10011=CARTESIAN_POINT('',(-3.465,-0.1,8.));
#10012=CARTESIAN_POINT('Origin',(-3.3,1.6,8.));
#10013=CARTESIAN_POINT('Origin',(-3.3,1.6,8.));
#10014=CARTESIAN_POINT('Origin',(2.02066721859313E-16,-0.1,11.3));
#10015=CARTESIAN_POINT('',(-0.165,0.,11.3));
#10016=CARTESIAN_POINT('Origin',(2.02066721859313E-16,0.,11.3));
#10017=CARTESIAN_POINT('',(-0.165,1.6,11.3));
#10018=CARTESIAN_POINT('',(-0.165,-0.1,11.3));
#10019=CARTESIAN_POINT('Origin',(2.02066721859313E-16,1.6,11.3));
#10020=CARTESIAN_POINT('Origin',(1.94289029309402E-16,1.6,11.3));
#10021=CARTESIAN_POINT('Origin',(3.3,-0.1,8.));
#10022=CARTESIAN_POINT('',(3.135,0.,8.));
#10023=CARTESIAN_POINT('Origin',(3.3,0.,8.));
#10024=CARTESIAN_POINT('',(3.135,1.6,8.));
#10025=CARTESIAN_POINT('',(3.135,-0.1,8.));
#10026=CARTESIAN_POINT('Origin',(3.3,1.6,8.));
#10027=CARTESIAN_POINT('Origin',(3.3,1.6,8.));
#10028=CARTESIAN_POINT('Origin',(-6.0620016557794E-16,-0.1,4.7));
#10029=CARTESIAN_POINT('',(-0.165000000000001,0.,4.7));
#10030=CARTESIAN_POINT('Origin',(-6.0620016557794E-16,0.,4.7));
#10031=CARTESIAN_POINT('',(-0.165000000000001,1.6,4.7));
#10032=CARTESIAN_POINT('',(-0.165000000000001,-0.1,4.7));
#10033=CARTESIAN_POINT('Origin',(-6.0620016557794E-16,1.6,4.7));
#10034=CARTESIAN_POINT('Origin',(-6.10622663543836E-16,1.6,4.7));
#10035=CARTESIAN_POINT('Origin',(4.4,1.,2.5));
#10036=CARTESIAN_POINT('',(4.73166247903554,0.5,4.8));
#10037=CARTESIAN_POINT('',(4.73166247903554,0.5,2.5));
#10038=CARTESIAN_POINT('',(4.73166247903554,0.5,2.5));
#10039=CARTESIAN_POINT('',(4.73166247903554,1.5,4.8));
#10040=CARTESIAN_POINT('Origin',(4.4,1.,4.8));
#10041=CARTESIAN_POINT('',(4.73166247903554,1.5,2.5));
#10042=CARTESIAN_POINT('',(4.73166247903554,1.5,2.5));
#10043=CARTESIAN_POINT('Origin',(4.4,1.,2.5));
#10044=CARTESIAN_POINT('Origin',(4.4,1.,2.5));
#10045=CARTESIAN_POINT('',(4.06833752096446,0.5,2.5));
#10046=CARTESIAN_POINT('',(4.06833752096446,0.5,4.8));
#10047=CARTESIAN_POINT('',(4.06833752096446,0.5,2.5));
#10048=CARTESIAN_POINT('',(4.06833752096446,1.5,2.5));
#10049=CARTESIAN_POINT('Origin',(4.4,1.,2.5));
#10050=CARTESIAN_POINT('',(4.06833752096446,1.5,4.8));
#10051=CARTESIAN_POINT('',(4.06833752096446,1.5,2.5));
#10052=CARTESIAN_POINT('Origin',(4.4,1.,4.8));
#10053=CARTESIAN_POINT('Origin',(4.4,1.,2.5));
#10054=CARTESIAN_POINT('',(2.2,0.5,2.5));
#10055=CARTESIAN_POINT('',(2.2,1.5,2.5));
#10056=CARTESIAN_POINT('',(4.07,1.,2.5));
#10057=CARTESIAN_POINT('Origin',(4.4,1.,2.5));
#10058=CARTESIAN_POINT('Origin',(-4.4,5.,2.5));
#10059=CARTESIAN_POINT('',(-4.06833752096446,4.5,4.8));
#10060=CARTESIAN_POINT('',(-4.06833752096446,4.5,2.5));
#10061=CARTESIAN_POINT('',(-4.06833752096446,4.5,2.5));
#10062=CARTESIAN_POINT('',(-4.06833752096446,5.5,4.8));
#10063=CARTESIAN_POINT('Origin',(-4.4,5.,4.8));
#10064=CARTESIAN_POINT('',(-4.06833752096446,5.5,2.5));
#10065=CARTESIAN_POINT('',(-4.06833752096446,5.5,2.5));
#10066=CARTESIAN_POINT('Origin',(-4.4,5.,2.5));
#10067=CARTESIAN_POINT('Origin',(-4.4,5.,2.5));
#10068=CARTESIAN_POINT('',(-4.73166247903554,4.5,2.5));
#10069=CARTESIAN_POINT('',(-4.73166247903554,4.5,4.8));
#10070=CARTESIAN_POINT('',(-4.73166247903554,4.5,2.5));
#10071=CARTESIAN_POINT('',(-4.73166247903554,5.5,2.5));
#10072=CARTESIAN_POINT('Origin',(-4.4,5.,2.5));
#10073=CARTESIAN_POINT('',(-4.73166247903554,5.5,4.8));
#10074=CARTESIAN_POINT('',(-4.73166247903554,5.5,2.5));
#10075=CARTESIAN_POINT('Origin',(-4.4,5.,4.8));
#10076=CARTESIAN_POINT('Origin',(-4.4,5.,2.5));
#10077=CARTESIAN_POINT('',(-2.2,4.5,2.5));
#10078=CARTESIAN_POINT('',(-2.2,5.5,2.5));
#10079=CARTESIAN_POINT('',(-4.73,5.,2.5));
#10080=CARTESIAN_POINT('Origin',(-4.4,5.,2.5));
#10081=CARTESIAN_POINT('Origin',(-4.4,1.,2.5));
#10082=CARTESIAN_POINT('',(-4.06833752096446,0.5,4.8));
#10083=CARTESIAN_POINT('',(-4.06833752096446,0.5,2.5));
#10084=CARTESIAN_POINT('',(-4.06833752096446,0.5,2.5));
#10085=CARTESIAN_POINT('',(-4.06833752096446,1.5,4.8));
#10086=CARTESIAN_POINT('Origin',(-4.4,1.,4.8));
#10087=CARTESIAN_POINT('',(-4.06833752096446,1.5,2.5));
#10088=CARTESIAN_POINT('',(-4.06833752096446,1.5,2.5));
#10089=CARTESIAN_POINT('Origin',(-4.4,1.,2.5));
#10090=CARTESIAN_POINT('Origin',(-4.4,1.,2.5));
#10091=CARTESIAN_POINT('',(-4.73166247903554,0.5,2.5));
#10092=CARTESIAN_POINT('',(-4.73166247903554,0.5,4.8));
#10093=CARTESIAN_POINT('',(-4.73166247903554,0.5,2.5));
#10094=CARTESIAN_POINT('',(-4.73166247903554,1.5,2.5));
#10095=CARTESIAN_POINT('Origin',(-4.4,1.,2.5));
#10096=CARTESIAN_POINT('',(-4.73166247903554,1.5,4.8));
#10097=CARTESIAN_POINT('',(-4.73166247903554,1.5,2.5));
#10098=CARTESIAN_POINT('Origin',(-4.4,1.,4.8));
#10099=CARTESIAN_POINT('Origin',(-4.4,1.,2.5));
#10100=CARTESIAN_POINT('',(-2.2,0.5,2.5));
#10101=CARTESIAN_POINT('',(-2.2,1.5,2.5));
#10102=CARTESIAN_POINT('',(-4.73,1.,2.5));
#10103=CARTESIAN_POINT('Origin',(-4.4,1.,2.5));
#10104=CARTESIAN_POINT('Origin',(4.4,5.,2.5));
#10105=CARTESIAN_POINT('',(4.73166247903554,4.5,4.8));
#10106=CARTESIAN_POINT('',(4.73166247903554,4.5,2.5));
#10107=CARTESIAN_POINT('',(4.73166247903554,4.5,2.5));
#10108=CARTESIAN_POINT('',(4.73166247903554,5.5,4.8));
#10109=CARTESIAN_POINT('Origin',(4.4,5.,4.8));
#10110=CARTESIAN_POINT('',(4.73166247903554,5.5,2.5));
#10111=CARTESIAN_POINT('',(4.73166247903554,5.5,2.5));
#10112=CARTESIAN_POINT('Origin',(4.4,5.,2.5));
#10113=CARTESIAN_POINT('Origin',(4.4,5.,2.5));
#10114=CARTESIAN_POINT('',(4.06833752096446,4.5,2.5));
#10115=CARTESIAN_POINT('',(4.06833752096446,4.5,4.8));
#10116=CARTESIAN_POINT('',(4.06833752096446,4.5,2.5));
#10117=CARTESIAN_POINT('',(4.06833752096446,5.5,2.5));
#10118=CARTESIAN_POINT('Origin',(4.4,5.,2.5));
#10119=CARTESIAN_POINT('',(4.06833752096446,5.5,4.8));
#10120=CARTESIAN_POINT('',(4.06833752096446,5.5,2.5));
#10121=CARTESIAN_POINT('Origin',(4.4,5.,4.8));
#10122=CARTESIAN_POINT('Origin',(4.4,5.,2.5));
#10123=CARTESIAN_POINT('',(2.2,4.5,2.5));
#10124=CARTESIAN_POINT('',(2.2,5.5,2.5));
#10125=CARTESIAN_POINT('',(4.07,5.,2.5));
#10126=CARTESIAN_POINT('Origin',(4.4,5.,2.5));
#10127=CARTESIAN_POINT('Origin',(-5.2,0.5,4.8));
#10128=CARTESIAN_POINT('',(5.2,0.5,4.8));
#10129=CARTESIAN_POINT('',(5.2,0.5,4.8));
#10130=CARTESIAN_POINT('',(5.2,1.5,4.8));
#10131=CARTESIAN_POINT('',(5.2,0.5,4.8));
#10132=CARTESIAN_POINT('',(5.2,1.5,4.8));
#10133=CARTESIAN_POINT('Origin',(-5.2,0.5,4.8));
#10134=CARTESIAN_POINT('',(2.4,1.5,4.8));
#10135=CARTESIAN_POINT('',(5.2,1.5,4.8));
#10136=CARTESIAN_POINT('',(2.4,0.5,4.8));
#10137=CARTESIAN_POINT('',(2.4,0.,4.8));
#10138=CARTESIAN_POINT('',(5.2,0.5,4.8));
#10139=CARTESIAN_POINT('Origin',(-5.2,4.5,4.8));
#10140=CARTESIAN_POINT('',(-2.4,4.5,4.8));
#10141=CARTESIAN_POINT('',(5.2,4.5,4.8));
#10142=CARTESIAN_POINT('',(-2.4,5.5,4.8));
#10143=CARTESIAN_POINT('',(-2.4,0.,4.8));
#10144=CARTESIAN_POINT('',(5.2,5.5,4.8));
#10145=CARTESIAN_POINT('Origin',(-5.2,4.5,4.8));
#10146=CARTESIAN_POINT('',(-5.2,5.5,4.8));
#10147=CARTESIAN_POINT('',(5.2,5.5,4.8));
#10148=CARTESIAN_POINT('',(-5.2,4.5,4.8));
#10149=CARTESIAN_POINT('',(-5.2,4.5,4.8));
#10150=CARTESIAN_POINT('',(5.2,4.5,4.8));
#10151=CARTESIAN_POINT('Origin',(0.,1.5,2.9));
#10152=CARTESIAN_POINT('',(5.2,1.5,1.));
#10153=CARTESIAN_POINT('',(5.2,1.5,1.));
#10154=CARTESIAN_POINT('',(-5.2,1.5,1.));
#10155=CARTESIAN_POINT('',(-5.2,1.5,1.));
#10156=CARTESIAN_POINT('',(-5.2,1.5,4.8));
#10157=CARTESIAN_POINT('',(-5.2,1.5,4.8));
#10158=CARTESIAN_POINT('',(5.2,1.5,4.8));
#10159=CARTESIAN_POINT('',(-2.4,1.5,4.8));
#10160=CARTESIAN_POINT('',(5.2,1.5,4.8));
#10161=CARTESIAN_POINT('Origin',(0.,1.5,8.));
#10162=CARTESIAN_POINT('Origin',(-5.2,0.5,4.8));
#10163=CARTESIAN_POINT('',(-2.4,0.5,4.8));
#10164=CARTESIAN_POINT('',(5.2,0.5,4.8));
#10165=CARTESIAN_POINT('',(-2.4,0.,4.8));
#10166=CARTESIAN_POINT('Origin',(-5.2,0.5,4.8));
#10167=CARTESIAN_POINT('',(-5.2,0.5,4.8));
#10168=CARTESIAN_POINT('',(-5.2,0.5,4.8));
#10169=CARTESIAN_POINT('',(5.2,0.5,4.8));
#10170=CARTESIAN_POINT('Origin',(0.,5.5,2.9));
#10171=CARTESIAN_POINT('',(2.4,5.5,4.8));
#10172=CARTESIAN_POINT('Origin',(0.,5.5,8.));
#10173=CARTESIAN_POINT('',(5.2,5.5,4.8));
#10174=CARTESIAN_POINT('',(5.2,5.5,4.8));
#10175=CARTESIAN_POINT('',(5.2,5.5,4.8));
#10176=CARTESIAN_POINT('',(5.2,5.5,1.));
#10177=CARTESIAN_POINT('',(5.2,5.5,1.));
#10178=CARTESIAN_POINT('',(-5.2,5.5,1.));
#10179=CARTESIAN_POINT('',(-5.2,5.5,1.));
#10180=CARTESIAN_POINT('',(-5.2,5.5,4.8));
#10181=CARTESIAN_POINT('Origin',(-5.2,4.5,4.8));
#10182=CARTESIAN_POINT('',(5.2,4.5,4.8));
#10183=CARTESIAN_POINT('',(5.2,4.5,4.8));
#10184=CARTESIAN_POINT('',(5.2,4.5,4.8));
#10185=CARTESIAN_POINT('Origin',(-5.2,4.5,4.8));
#10186=CARTESIAN_POINT('',(2.4,4.5,4.8));
#10187=CARTESIAN_POINT('',(2.4,0.,4.8));
#10188=CARTESIAN_POINT('',(5.2,4.5,4.8));
#10189=CARTESIAN_POINT('Origin',(4.4,1.,0.9));
#10190=CARTESIAN_POINT('',(4.07,1.,1.));
#10191=CARTESIAN_POINT('Origin',(4.4,1.,1.));
#10192=CARTESIAN_POINT('',(4.07,1.,0.9));
#10193=CARTESIAN_POINT('Origin',(-4.4,5.,0.9));
#10194=CARTESIAN_POINT('',(-4.73,5.,1.));
#10195=CARTESIAN_POINT('Origin',(-4.4,5.,1.));
#10196=CARTESIAN_POINT('',(-4.73,5.,0.9));
#10197=CARTESIAN_POINT('Origin',(-4.4,1.,0.9));
#10198=CARTESIAN_POINT('',(-4.73,1.,1.));
#10199=CARTESIAN_POINT('Origin',(-4.4,1.,1.));
#10200=CARTESIAN_POINT('',(-4.73,1.,0.9));
#10201=CARTESIAN_POINT('Origin',(4.4,5.,0.9));
#10202=CARTESIAN_POINT('',(4.07,5.,1.));
#10203=CARTESIAN_POINT('Origin',(4.4,5.,1.));
#10204=CARTESIAN_POINT('',(4.07,5.,0.9));
#10205=CARTESIAN_POINT('Origin',(-5.2,4.5,1.));
#10206=CARTESIAN_POINT('',(-5.2,4.5,1.));
#10207=CARTESIAN_POINT('',(-5.2,4.5,4.8));
#10208=CARTESIAN_POINT('',(-5.2,4.5,1.));
#10209=CARTESIAN_POINT('Origin',(5.2,4.5,1.));
#10210=CARTESIAN_POINT('',(5.2,4.5,1.));
#10211=CARTESIAN_POINT('',(-5.2,4.5,1.));
#10212=CARTESIAN_POINT('',(5.2,4.5,1.));
#10213=CARTESIAN_POINT('Origin',(5.2,4.5,4.8));
#10214=CARTESIAN_POINT('',(5.2,4.5,1.));
#10215=CARTESIAN_POINT('Origin',(0.,4.5,2.9));
#10216=CARTESIAN_POINT('Origin',(0.,4.5,8.));
#10217=CARTESIAN_POINT('Origin',(-5.2,0.5,1.));
#10218=CARTESIAN_POINT('',(-5.2,0.5,1.));
#10219=CARTESIAN_POINT('',(-5.2,0.5,4.8));
#10220=CARTESIAN_POINT('',(-5.2,0.5,1.));
#10221=CARTESIAN_POINT('Origin',(5.2,0.5,1.));
#10222=CARTESIAN_POINT('',(5.2,0.5,1.));
#10223=CARTESIAN_POINT('',(-5.2,0.5,1.));
#10224=CARTESIAN_POINT('',(5.2,0.5,1.));
#10225=CARTESIAN_POINT('Origin',(5.2,0.5,4.8));
#10226=CARTESIAN_POINT('',(5.2,0.5,1.));
#10227=CARTESIAN_POINT('Origin',(0.,0.5,2.9));
#10228=CARTESIAN_POINT('Origin',(0.,0.5,8.));
#10229=CARTESIAN_POINT('Origin',(0.,0.,8.));
#10230=CARTESIAN_POINT('',(-2.6,6.,8.));
#10231=CARTESIAN_POINT('Origin',(0.,6.,8.));
#10232=CARTESIAN_POINT('',(-2.6,0.,8.));
#10233=CARTESIAN_POINT('',(-2.6,0.,8.));
#10234=CARTESIAN_POINT('Origin',(0.,0.,8.));
#10235=CARTESIAN_POINT('Origin',(0.,0.,8.));
#10236=CARTESIAN_POINT('',(-4.,6.,8.));
#10237=CARTESIAN_POINT('Origin',(0.,6.,8.));
#10238=CARTESIAN_POINT('',(-4.,0.,8.));
#10239=CARTESIAN_POINT('',(-4.,0.,8.));
#10240=CARTESIAN_POINT('Origin',(0.,0.,8.));
#10241=CARTESIAN_POINT('Origin',(0.,6.,8.));
#10242=CARTESIAN_POINT('Origin',(0.,0.,8.));
#12699=UNCERTAINTY_MEASURE_WITH_UNIT(LENGTH_MEASURE(0.001),#12784,
'DISTANCE_ACCURACY_VALUE',
'Maximum model space distance between geometric entities at asserted c
onnectivities');
#12739=UNCERTAINTY_MEASURE_WITH_UNIT(LENGTH_MEASURE(0.001),#12784,
'DISTANCE_ACCURACY_VALUE',
'Maximum model space distance between geometric entities at asserted c
onnectivities');
#12743=(
GEOMETRIC_REPRESENTATION_CONTEXT(3)
GLOBAL_UNCERTAINTY_ASSIGNED_CONTEXT((#12699))
GLOBAL_UNIT_ASSIGNED_CONTEXT((#12784,#12786,#12787))
REPRESENTATION_CONTEXT('','3D')
);
#12783=(
GEOMETRIC_REPRESENTATION_CONTEXT(3)
GLOBAL_UNCERTAINTY_ASSIGNED_CONTEXT((#12739))
GLOBAL_UNIT_ASSIGNED_CONTEXT((#12784,#12786,#12787))
REPRESENTATION_CONTEXT('','3D')
);
#12784=(
LENGTH_UNIT()
NAMED_UNIT(*)
SI_UNIT(.CENTI.,.METRE.)
);
#12786=(
NAMED_UNIT(*)
PLANE_ANGLE_UNIT()
SI_UNIT($,.RADIAN.)
);
#12787=(
NAMED_UNIT(*)
SI_UNIT($,.STERADIAN.)
SOLID_ANGLE_UNIT()
);
#12791=SHAPE_DEFINITION_REPRESENTATION(#12834,#12934);
#12834=PRODUCT_DEFINITION_SHAPE('',$,#12978);
#12934=SHAPE_REPRESENTATION('',(#6981),#12743);
#12974=PRODUCT_DEFINITION_CONTEXT('part definition',#13105,'design');
#12978=PRODUCT_DEFINITION('Bearing housing','Bearing housing',#13021,#12974);
#13021=PRODUCT_DEFINITION_FORMATION('',$,#13110);
#13105=APPLICATION_CONTEXT(
'Core Data for Automotive Mechanical Design Process');
#13106=PRODUCT_CONTEXT('part definition',#13105,'mechanical');
#13110=PRODUCT('Bearing housing','Bearing housing','Bearing housing',(#13106));
#13206=COLOUR_RGB('Grey',0.48,0.52,0.57);
#13207=FILL_AREA_STYLE_COLOUR('',#13206);
#13208=FILL_AREA_STYLE('',(#13207));
#13209=SURFACE_STYLE_FILL_AREA(#13208);
#13210=SURFACE_SIDE_STYLE('',(#13209));
#13211=SURFACE_STYLE_USAGE(.BOTH.,#13210);
#13212=PRESENTATION_STYLE_ASSIGNMENT((#13211));
ENDSEC;
END-ISO-10303-21;
